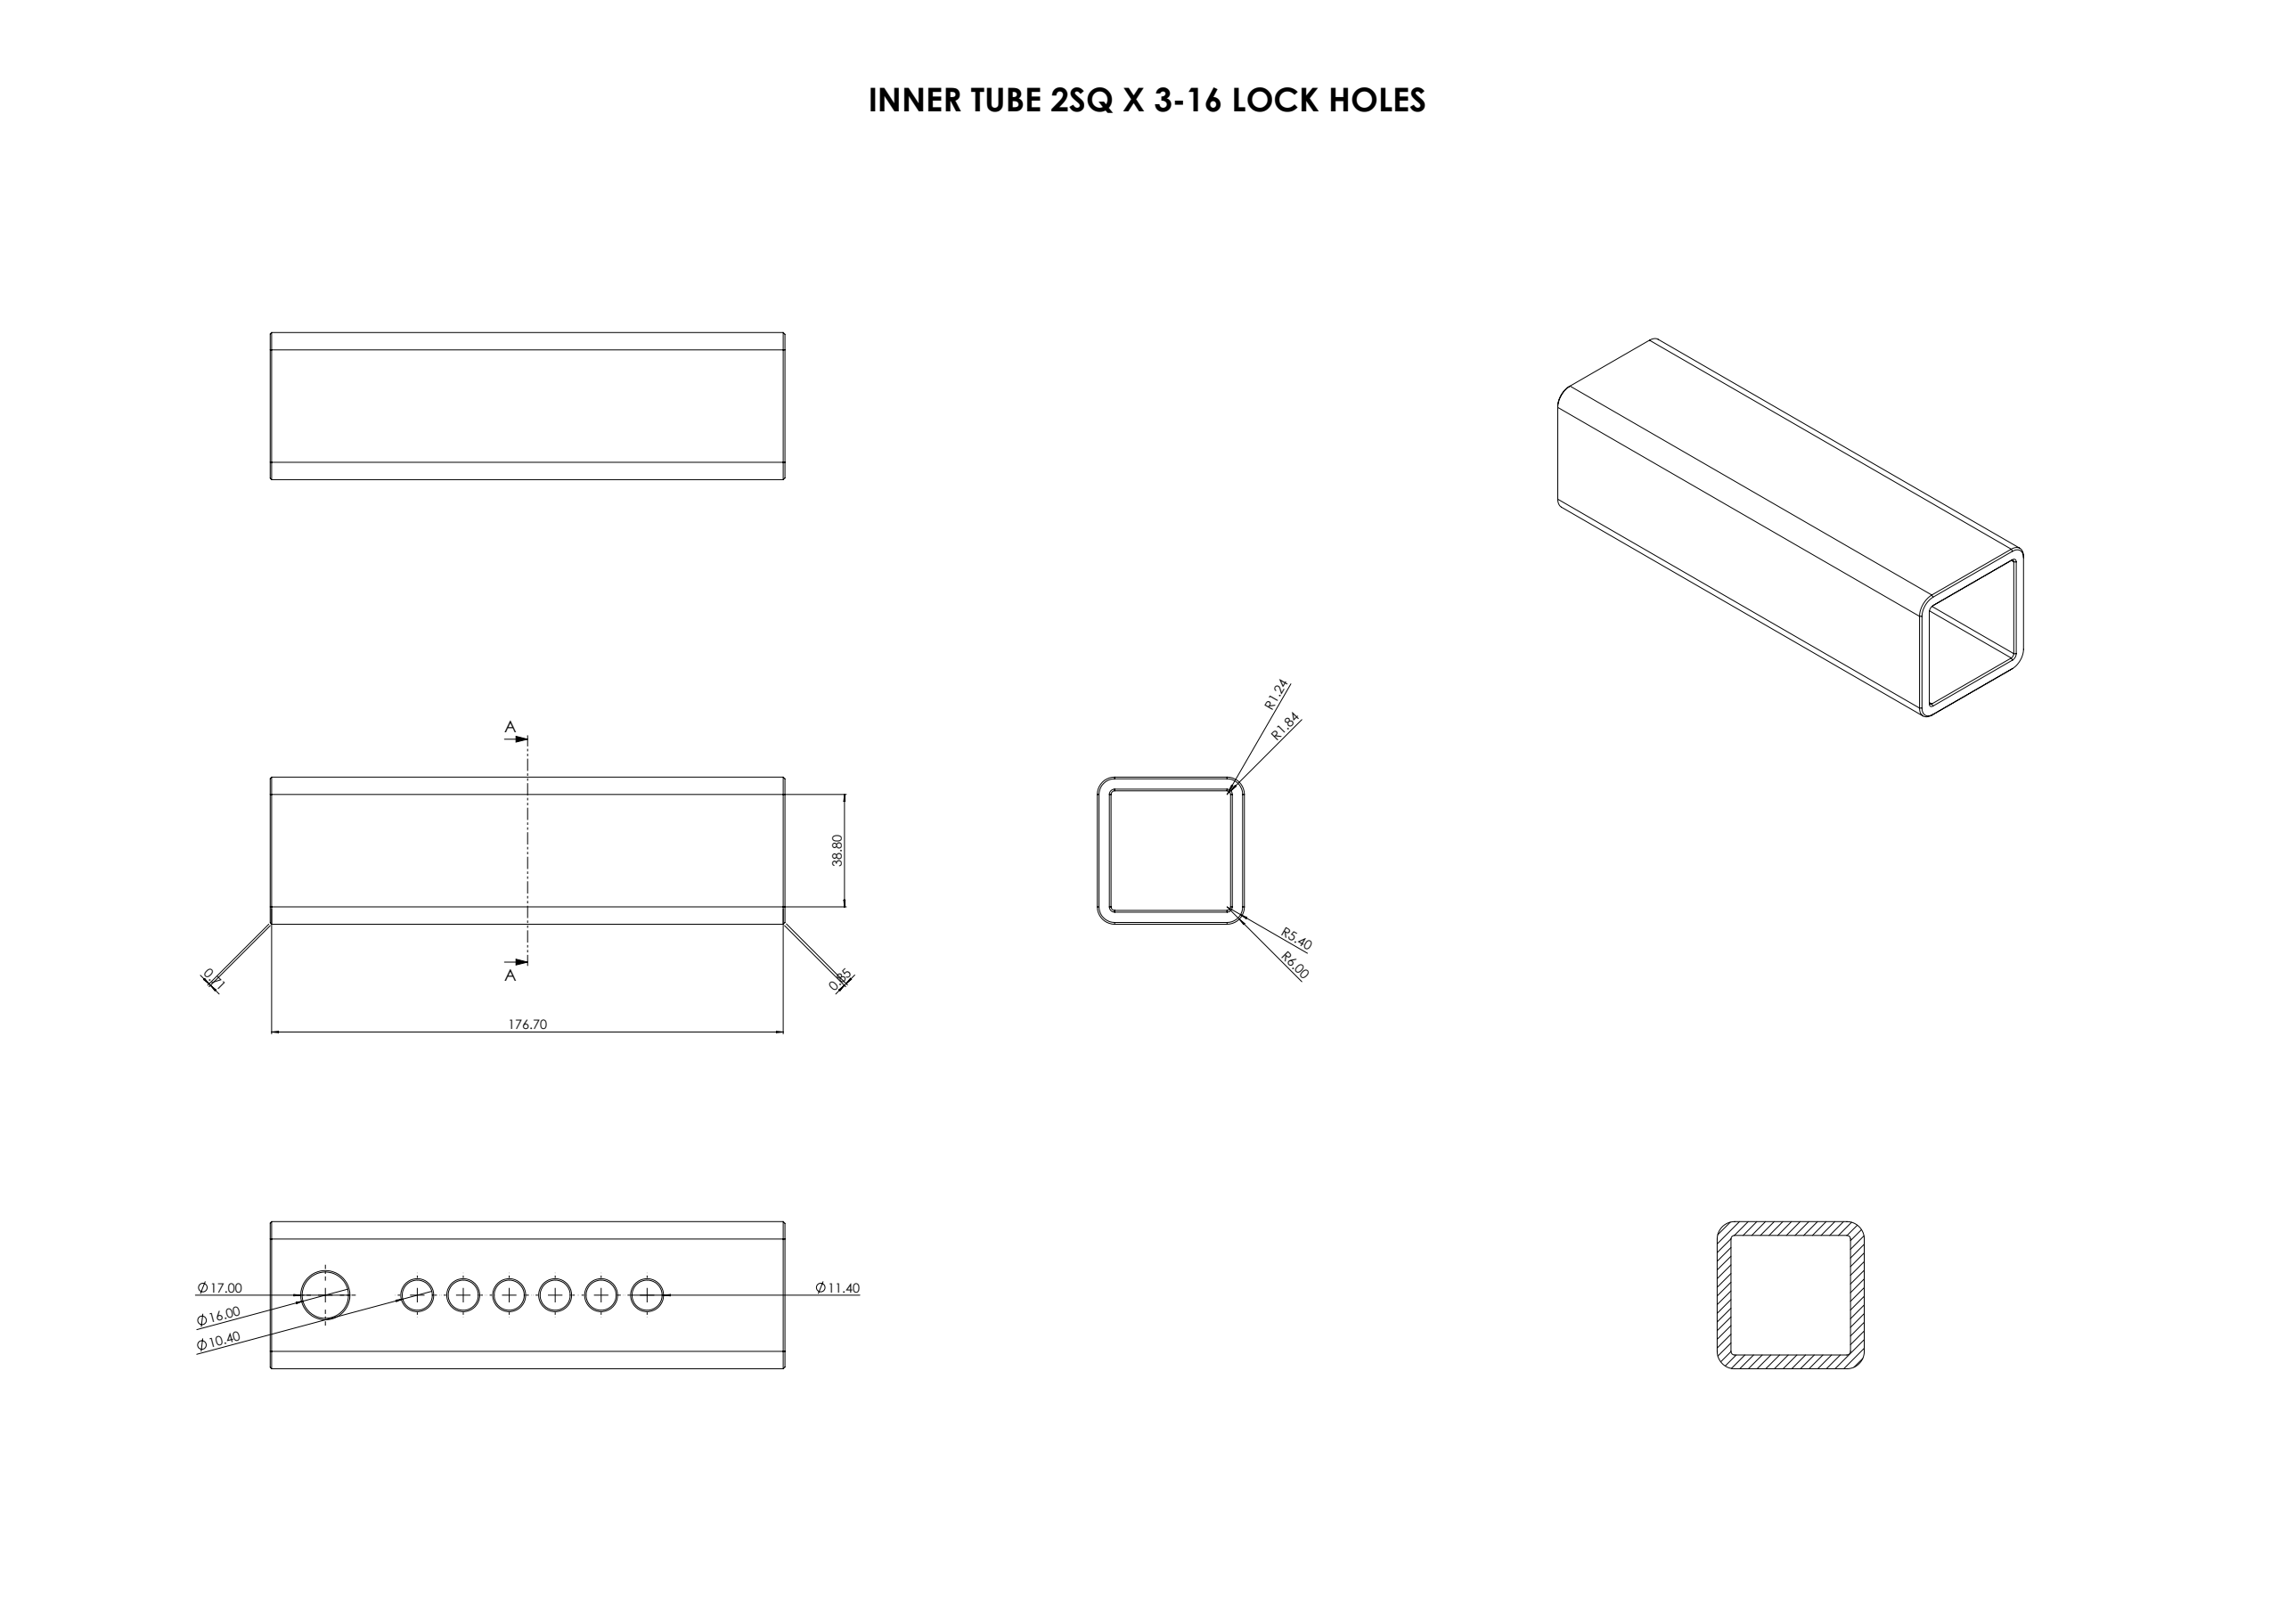
ISO-10303-21;
HEADER;
/* Generated by software containing ST-Developer
 * from STEP Tools, Inc. (www.steptools.com) 
 */

FILE_DESCRIPTION(
/* description */ (''),
/* implementation_level */ '2;1');

FILE_NAME(
/* name */ '05_Inner_Tube_2sq_x_3-16_Lock_Holes.step',
/* time_stamp */ '2026-10-25T01:30:15-07:00',
/* author */ (''),
/* organization */ (''),
/* preprocessor_version */ 'ST-DEVELOPER v20.2',
/* originating_system */ 'Autodesk Translation Framework v15.15.0.0',
/* authorisation */ '');

FILE_SCHEMA (('AUTOMOTIVE_DESIGN { 1 0 10303 214 3 1 1 }'));
ENDSEC;

DATA;
#10=MECHANICAL_DESIGN_GEOMETRIC_PRESENTATION_REPRESENTATION('',(#567),#32309);
#539=SHAPE_REPRESENTATION_RELATIONSHIP('SRR','None',#32366,#553);
#553=ADVANCED_BREP_SHAPE_REPRESENTATION('',(#581),#32299);
#567=STYLED_ITEM('',(#32488),#581);
#581=MANIFOLD_SOLID_BREP('Body1',#13808);
#599=FACE_BOUND('',#2235,.T.);
#600=FACE_BOUND('',#2236,.T.);
#601=FACE_BOUND('',#2237,.T.);
#602=FACE_BOUND('',#2238,.T.);
#603=FACE_BOUND('',#2239,.T.);
#604=FACE_BOUND('',#2240,.T.);
#605=FACE_BOUND('',#2254,.T.);
#606=FACE_BOUND('',#2255,.T.);
#607=FACE_BOUND('',#2256,.T.);
#608=FACE_BOUND('',#2257,.T.);
#609=FACE_BOUND('',#2258,.T.);
#610=FACE_BOUND('',#2259,.T.);
#611=FACE_BOUND('',#2260,.T.);
#612=FACE_BOUND('',#2273,.T.);
#613=FACE_BOUND('',#2288,.T.);
#614=FACE_BOUND('',#2289,.T.);
#615=FACE_BOUND('',#2290,.T.);
#616=FACE_BOUND('',#2291,.T.);
#617=FACE_BOUND('',#2292,.T.);
#618=FACE_BOUND('',#2293,.T.);
#619=FACE_BOUND('',#2294,.T.);
#620=FACE_BOUND('',#2312,.T.);
#621=FACE_BOUND('',#2313,.T.);
#622=FACE_BOUND('',#2314,.T.);
#623=FACE_BOUND('',#2315,.T.);
#624=FACE_BOUND('',#2316,.T.);
#625=FACE_BOUND('',#2317,.T.);
#626=FACE_BOUND('',#2334,.T.);
#685=CYLINDRICAL_SURFACE('',#14214,5.2);
#686=CYLINDRICAL_SURFACE('',#14218,5.2);
#687=CYLINDRICAL_SURFACE('',#14222,5.2);
#688=CYLINDRICAL_SURFACE('',#14226,5.2);
#689=CYLINDRICAL_SURFACE('',#14230,5.2);
#690=CYLINDRICAL_SURFACE('',#14234,5.2);
#691=CYLINDRICAL_SURFACE('',#14246,5.2);
#692=CYLINDRICAL_SURFACE('',#14264,1.2375);
#693=CYLINDRICAL_SURFACE('',#14266,1.2375);
#694=CYLINDRICAL_SURFACE('',#14275,8.);
#695=CYLINDRICAL_SURFACE('',#14279,5.2);
#696=CYLINDRICAL_SURFACE('',#14283,5.2);
#697=CYLINDRICAL_SURFACE('',#14287,5.2);
#698=CYLINDRICAL_SURFACE('',#14291,5.2);
#699=CYLINDRICAL_SURFACE('',#14295,5.2);
#700=CYLINDRICAL_SURFACE('',#14324,6.00000000000001);
#701=CYLINDRICAL_SURFACE('',#14326,6.00000000000001);
#702=CYLINDRICAL_SURFACE('',#14355,6.00000000000001);
#703=CYLINDRICAL_SURFACE('',#14371,1.2375);
#704=CYLINDRICAL_SURFACE('',#14373,1.23749999999999);
#705=CYLINDRICAL_SURFACE('',#14376,6.00000000000001);
#855=CIRCLE('',#14206,5.69999999999999);
#856=CIRCLE('',#14207,5.2);
#857=CIRCLE('',#14209,5.7);
#858=CIRCLE('',#14210,5.7);
#859=CIRCLE('',#14211,5.69999999999999);
#860=CIRCLE('',#14212,5.7);
#861=CIRCLE('',#14213,5.7);
#862=CIRCLE('',#14215,5.2);
#863=CIRCLE('',#14217,5.2);
#864=CIRCLE('',#14219,5.2);
#865=CIRCLE('',#14221,5.2);
#866=CIRCLE('',#14223,5.2);
#867=CIRCLE('',#14225,5.2);
#868=CIRCLE('',#14227,5.2);
#869=CIRCLE('',#14229,5.2);
#870=CIRCLE('',#14231,5.2);
#871=CIRCLE('',#14233,5.2);
#872=CIRCLE('',#14235,5.2);
#873=CIRCLE('',#14237,5.69999999999999);
#874=CIRCLE('',#14238,5.2);
#875=CIRCLE('',#14240,5.7);
#876=CIRCLE('',#14241,5.7);
#877=CIRCLE('',#14242,5.69999999999999);
#878=CIRCLE('',#14243,5.7);
#879=CIRCLE('',#14244,5.7);
#880=CIRCLE('',#14245,8.5);
#881=CIRCLE('',#14247,5.2);
#882=CIRCLE('',#14250,1.2375);
#883=CIRCLE('',#14251,1.7375);
#884=CIRCLE('',#14254,1.23749999999999);
#885=CIRCLE('',#14255,1.7375);
#886=CIRCLE('',#14258,1.2375);
#887=CIRCLE('',#14259,1.7375);
#888=CIRCLE('',#14262,1.2375);
#889=CIRCLE('',#14263,1.7375);
#890=CIRCLE('',#14265,1.2375);
#891=CIRCLE('',#14267,1.2375);
#892=CIRCLE('',#14269,5.50000000000001);
#893=CIRCLE('',#14270,5.50000000000001);
#894=CIRCLE('',#14271,5.50000000000002);
#895=CIRCLE('',#14272,5.50000000000002);
#896=CIRCLE('',#14274,8.);
#897=CIRCLE('',#14276,8.);
#898=CIRCLE('',#14278,5.2);
#899=CIRCLE('',#14280,5.2);
#900=CIRCLE('',#14282,5.2);
#901=CIRCLE('',#14284,5.2);
#902=CIRCLE('',#14286,5.2);
#903=CIRCLE('',#14288,5.2);
#904=CIRCLE('',#14290,5.2);
#905=CIRCLE('',#14292,5.2);
#906=CIRCLE('',#14294,5.2);
#907=CIRCLE('',#14296,5.2);
#908=CIRCLE('',#14298,8.5);
#909=CIRCLE('',#14300,5.69999999999999);
#910=CIRCLE('',#14301,5.7);
#911=CIRCLE('',#14302,5.7);
#912=CIRCLE('',#14303,5.69999999999999);
#913=CIRCLE('',#14304,5.7);
#914=CIRCLE('',#14305,5.7);
#915=CIRCLE('',#14314,6.00000000000001);
#916=CIRCLE('',#14317,6.00000000000001);
#917=CIRCLE('',#14320,6.00000000000001);
#918=CIRCLE('',#14323,6.00000000000001);
#919=CIRCLE('',#14325,6.00000000000001);
#920=CIRCLE('',#14327,6.00000000000001);
#921=CIRCLE('',#14329,5.69999999999999);
#922=CIRCLE('',#14330,5.7);
#923=CIRCLE('',#14331,5.7);
#924=CIRCLE('',#14332,5.69999999999999);
#925=CIRCLE('',#14333,5.7);
#926=CIRCLE('',#14334,5.7);
#927=CIRCLE('',#14343,5.40000000000001);
#928=CIRCLE('',#14346,5.40000000000002);
#929=CIRCLE('',#14347,6.00000000000001);
#930=CIRCLE('',#14350,5.40000000000002);
#931=CIRCLE('',#14351,6.00000000000001);
#932=CIRCLE('',#14354,5.40000000000001);
#933=CIRCLE('',#14357,1.8375);
#934=CIRCLE('',#14358,1.8375);
#935=CIRCLE('',#14359,1.83749999999999);
#936=CIRCLE('',#14360,1.8375);
#937=CIRCLE('',#14365,1.2375);
#938=CIRCLE('',#14368,1.23749999999999);
#1135=CONICAL_SURFACE('',#14205,5.44999999999999,0.785398163397448);
#1136=CONICAL_SURFACE('',#14216,5.45,0.785398163397451);
#1137=CONICAL_SURFACE('',#14220,5.45,0.785398163397451);
#1138=CONICAL_SURFACE('',#14224,5.45,0.785398163397448);
#1139=CONICAL_SURFACE('',#14228,5.45,0.785398163397448);
#1140=CONICAL_SURFACE('',#14232,5.44999999999999,0.785398163397448);
#1141=CONICAL_SURFACE('',#14236,5.44999999999999,0.785398163397446);
#1142=CONICAL_SURFACE('',#14249,1.4875,0.785398163397449);
#1143=CONICAL_SURFACE('',#14253,1.48749999999999,0.785398163397452);
#1144=CONICAL_SURFACE('',#14257,1.4875,0.785398163397449);
#1145=CONICAL_SURFACE('',#14261,1.4875,0.785398163397449);
#1146=CONICAL_SURFACE('',#14273,8.25,0.785398163397446);
#1147=CONICAL_SURFACE('',#14277,5.45,0.785398163397446);
#1148=CONICAL_SURFACE('',#14281,5.45,0.785398163397446);
#1149=CONICAL_SURFACE('',#14285,5.45,0.785398163397448);
#1150=CONICAL_SURFACE('',#14289,5.45,0.785398163397448);
#1151=CONICAL_SURFACE('',#14293,5.44999999999999,0.785398163397446);
#1152=CONICAL_SURFACE('',#14297,8.25,0.785398163397446);
#1153=CONICAL_SURFACE('',#14306,5.44999999999999,0.785398163397446);
#1154=CONICAL_SURFACE('',#14307,5.45,0.785398163397446);
#1155=CONICAL_SURFACE('',#14308,5.45,0.785398163397446);
#1156=CONICAL_SURFACE('',#14309,5.45,0.785398163397448);
#1157=CONICAL_SURFACE('',#14310,5.45,0.785398163397448);
#1158=CONICAL_SURFACE('',#14311,5.44999999999999,0.785398163397446);
#1159=CONICAL_SURFACE('',#14313,5.75000000000002,0.785398163397449);
#1160=CONICAL_SURFACE('',#14316,5.75000000000002,0.785398163397449);
#1161=CONICAL_SURFACE('',#14319,5.75000000000001,0.785398163397451);
#1162=CONICAL_SURFACE('',#14322,5.75000000000001,0.785398163397449);
#1163=CONICAL_SURFACE('',#14335,5.44999999999999,0.785398163397448);
#1164=CONICAL_SURFACE('',#14336,5.45,0.785398163397448);
#1165=CONICAL_SURFACE('',#14337,5.45,0.785398163397448);
#1166=CONICAL_SURFACE('',#14338,5.45,0.785398163397451);
#1167=CONICAL_SURFACE('',#14339,5.45,0.785398163397451);
#1168=CONICAL_SURFACE('',#14340,5.44999999999999,0.785398163397448);
#1169=CONICAL_SURFACE('',#14342,5.70000000000001,0.785398163397431);
#1170=CONICAL_SURFACE('',#14345,5.70000000000002,0.785398163397426);
#1171=CONICAL_SURFACE('',#14349,5.70000000000002,0.785398163397426);
#1172=CONICAL_SURFACE('',#14353,5.70000000000001,0.785398163397431);
#1173=CONICAL_SURFACE('',#14362,1.5375,0.78539816339743);
#1174=CONICAL_SURFACE('',#14364,1.5375,0.78539816339743);
#1175=CONICAL_SURFACE('',#14367,1.53749999999999,0.785398163397429);
#1176=CONICAL_SURFACE('',#14370,1.5375,0.785398163397426);
#1426=FACE_OUTER_BOUND('',#2233,.T.);
#1427=FACE_OUTER_BOUND('',#2234,.T.);
#1428=FACE_OUTER_BOUND('',#2241,.T.);
#1429=FACE_OUTER_BOUND('',#2242,.T.);
#1430=FACE_OUTER_BOUND('',#2243,.T.);
#1431=FACE_OUTER_BOUND('',#2244,.T.);
#1432=FACE_OUTER_BOUND('',#2245,.T.);
#1433=FACE_OUTER_BOUND('',#2246,.T.);
#1434=FACE_OUTER_BOUND('',#2247,.T.);
#1435=FACE_OUTER_BOUND('',#2248,.T.);
#1436=FACE_OUTER_BOUND('',#2249,.T.);
#1437=FACE_OUTER_BOUND('',#2250,.T.);
#1438=FACE_OUTER_BOUND('',#2251,.T.);
#1439=FACE_OUTER_BOUND('',#2252,.T.);
#1440=FACE_OUTER_BOUND('',#2253,.T.);
#1441=FACE_OUTER_BOUND('',#2261,.T.);
#1442=FACE_OUTER_BOUND('',#2262,.T.);
#1443=FACE_OUTER_BOUND('',#2263,.T.);
#1444=FACE_OUTER_BOUND('',#2264,.T.);
#1445=FACE_OUTER_BOUND('',#2265,.T.);
#1446=FACE_OUTER_BOUND('',#2266,.T.);
#1447=FACE_OUTER_BOUND('',#2267,.T.);
#1448=FACE_OUTER_BOUND('',#2268,.T.);
#1449=FACE_OUTER_BOUND('',#2269,.T.);
#1450=FACE_OUTER_BOUND('',#2270,.T.);
#1451=FACE_OUTER_BOUND('',#2271,.T.);
#1452=FACE_OUTER_BOUND('',#2272,.T.);
#1453=FACE_OUTER_BOUND('',#2274,.T.);
#1454=FACE_OUTER_BOUND('',#2275,.T.);
#1455=FACE_OUTER_BOUND('',#2276,.T.);
#1456=FACE_OUTER_BOUND('',#2277,.T.);
#1457=FACE_OUTER_BOUND('',#2278,.T.);
#1458=FACE_OUTER_BOUND('',#2279,.T.);
#1459=FACE_OUTER_BOUND('',#2280,.T.);
#1460=FACE_OUTER_BOUND('',#2281,.T.);
#1461=FACE_OUTER_BOUND('',#2282,.T.);
#1462=FACE_OUTER_BOUND('',#2283,.T.);
#1463=FACE_OUTER_BOUND('',#2284,.T.);
#1464=FACE_OUTER_BOUND('',#2285,.T.);
#1465=FACE_OUTER_BOUND('',#2286,.T.);
#1466=FACE_OUTER_BOUND('',#2287,.T.);
#1467=FACE_OUTER_BOUND('',#2295,.T.);
#1468=FACE_OUTER_BOUND('',#2296,.T.);
#1469=FACE_OUTER_BOUND('',#2297,.T.);
#1470=FACE_OUTER_BOUND('',#2298,.T.);
#1471=FACE_OUTER_BOUND('',#2299,.T.);
#1472=FACE_OUTER_BOUND('',#2300,.T.);
#1473=FACE_OUTER_BOUND('',#2301,.T.);
#1474=FACE_OUTER_BOUND('',#2302,.T.);
#1475=FACE_OUTER_BOUND('',#2303,.T.);
#1476=FACE_OUTER_BOUND('',#2304,.T.);
#1477=FACE_OUTER_BOUND('',#2305,.T.);
#1478=FACE_OUTER_BOUND('',#2306,.T.);
#1479=FACE_OUTER_BOUND('',#2307,.T.);
#1480=FACE_OUTER_BOUND('',#2308,.T.);
#1481=FACE_OUTER_BOUND('',#2309,.T.);
#1482=FACE_OUTER_BOUND('',#2310,.T.);
#1483=FACE_OUTER_BOUND('',#2311,.T.);
#1484=FACE_OUTER_BOUND('',#2318,.T.);
#1485=FACE_OUTER_BOUND('',#2319,.T.);
#1486=FACE_OUTER_BOUND('',#2320,.T.);
#1487=FACE_OUTER_BOUND('',#2321,.T.);
#1488=FACE_OUTER_BOUND('',#2322,.T.);
#1489=FACE_OUTER_BOUND('',#2323,.T.);
#1490=FACE_OUTER_BOUND('',#2324,.T.);
#1491=FACE_OUTER_BOUND('',#2325,.T.);
#1492=FACE_OUTER_BOUND('',#2326,.T.);
#1493=FACE_OUTER_BOUND('',#2327,.T.);
#1494=FACE_OUTER_BOUND('',#2328,.T.);
#1495=FACE_OUTER_BOUND('',#2329,.T.);
#1496=FACE_OUTER_BOUND('',#2330,.T.);
#1497=FACE_OUTER_BOUND('',#2331,.T.);
#1498=FACE_OUTER_BOUND('',#2332,.T.);
#1499=FACE_OUTER_BOUND('',#2333,.T.);
#1500=FACE_OUTER_BOUND('',#2335,.T.);
#1501=FACE_OUTER_BOUND('',#2336,.T.);
#1502=FACE_OUTER_BOUND('',#2337,.T.);
#1503=FACE_OUTER_BOUND('',#2338,.T.);
#1504=FACE_OUTER_BOUND('',#2339,.T.);
#1505=FACE_OUTER_BOUND('',#2340,.T.);
#1506=FACE_OUTER_BOUND('',#2341,.T.);
#1507=FACE_OUTER_BOUND('',#2342,.T.);
#1508=FACE_OUTER_BOUND('',#2343,.T.);
#1509=FACE_OUTER_BOUND('',#2344,.T.);
#1510=FACE_OUTER_BOUND('',#2345,.T.);
#1511=FACE_OUTER_BOUND('',#2346,.T.);
#1512=FACE_OUTER_BOUND('',#2347,.T.);
#1513=FACE_OUTER_BOUND('',#2348,.T.);
#1514=FACE_OUTER_BOUND('',#2349,.T.);
#2233=EDGE_LOOP('',(#9555,#9556,#9557,#9558));
#2234=EDGE_LOOP('',(#9559,#9560,#9561,#9562));
#2235=EDGE_LOOP('',(#9563));
#2236=EDGE_LOOP('',(#9564));
#2237=EDGE_LOOP('',(#9565));
#2238=EDGE_LOOP('',(#9566));
#2239=EDGE_LOOP('',(#9567));
#2240=EDGE_LOOP('',(#9568));
#2241=EDGE_LOOP('',(#9569,#9570,#9571,#9572));
#2242=EDGE_LOOP('',(#9573,#9574,#9575,#9576));
#2243=EDGE_LOOP('',(#9577,#9578,#9579,#9580));
#2244=EDGE_LOOP('',(#9581,#9582,#9583,#9584));
#2245=EDGE_LOOP('',(#9585,#9586,#9587,#9588));
#2246=EDGE_LOOP('',(#9589,#9590,#9591,#9592));
#2247=EDGE_LOOP('',(#9593,#9594,#9595,#9596));
#2248=EDGE_LOOP('',(#9597,#9598,#9599,#9600));
#2249=EDGE_LOOP('',(#9601,#9602,#9603,#9604));
#2250=EDGE_LOOP('',(#9605,#9606,#9607,#9608));
#2251=EDGE_LOOP('',(#9609,#9610,#9611,#9612));
#2252=EDGE_LOOP('',(#9613,#9614,#9615,#9616));
#2253=EDGE_LOOP('',(#9617,#9618,#9619,#9620));
#2254=EDGE_LOOP('',(#9621));
#2255=EDGE_LOOP('',(#9622));
#2256=EDGE_LOOP('',(#9623));
#2257=EDGE_LOOP('',(#9624));
#2258=EDGE_LOOP('',(#9625));
#2259=EDGE_LOOP('',(#9626));
#2260=EDGE_LOOP('',(#9627));
#2261=EDGE_LOOP('',(#9628,#9629,#9630,#9631));
#2262=EDGE_LOOP('',(#9632,#9633,#9634,#9635));
#2263=EDGE_LOOP('',(#9636,#9637,#9638,#9639));
#2264=EDGE_LOOP('',(#9640,#9641,#9642,#9643));
#2265=EDGE_LOOP('',(#9644,#9645,#9646,#9647));
#2266=EDGE_LOOP('',(#9648,#9649,#9650,#9651));
#2267=EDGE_LOOP('',(#9652,#9653,#9654,#9655));
#2268=EDGE_LOOP('',(#9656,#9657,#9658,#9659));
#2269=EDGE_LOOP('',(#9660,#9661,#9662,#9663));
#2270=EDGE_LOOP('',(#9664,#9665,#9666,#9667));
#2271=EDGE_LOOP('',(#9668,#9669,#9670,#9671));
#2272=EDGE_LOOP('',(#9672,#9673,#9674,#9675,#9676,#9677,#9678,#9679));
#2273=EDGE_LOOP('',(#9680,#9681,#9682,#9683,#9684,#9685,#9686,#9687));
#2274=EDGE_LOOP('',(#9688,#9689,#9690,#9691));
#2275=EDGE_LOOP('',(#9692,#9693,#9694,#9695));
#2276=EDGE_LOOP('',(#9696,#9697,#9698,#9699));
#2277=EDGE_LOOP('',(#9700,#9701,#9702,#9703));
#2278=EDGE_LOOP('',(#9704,#9705,#9706,#9707));
#2279=EDGE_LOOP('',(#9708,#9709,#9710,#9711));
#2280=EDGE_LOOP('',(#9712,#9713,#9714,#9715));
#2281=EDGE_LOOP('',(#9716,#9717,#9718,#9719));
#2282=EDGE_LOOP('',(#9720,#9721,#9722,#9723));
#2283=EDGE_LOOP('',(#9724,#9725,#9726,#9727));
#2284=EDGE_LOOP('',(#9728,#9729,#9730,#9731));
#2285=EDGE_LOOP('',(#9732,#9733,#9734,#9735));
#2286=EDGE_LOOP('',(#9736,#9737,#9738,#9739));
#2287=EDGE_LOOP('',(#9740,#9741,#9742,#9743));
#2288=EDGE_LOOP('',(#9744));
#2289=EDGE_LOOP('',(#9745));
#2290=EDGE_LOOP('',(#9746));
#2291=EDGE_LOOP('',(#9747));
#2292=EDGE_LOOP('',(#9748));
#2293=EDGE_LOOP('',(#9749));
#2294=EDGE_LOOP('',(#9750));
#2295=EDGE_LOOP('',(#9751,#9752,#9753,#9754));
#2296=EDGE_LOOP('',(#9755,#9756,#9757,#9758));
#2297=EDGE_LOOP('',(#9759,#9760,#9761,#9762));
#2298=EDGE_LOOP('',(#9763,#9764,#9765,#9766));
#2299=EDGE_LOOP('',(#9767,#9768,#9769,#9770));
#2300=EDGE_LOOP('',(#9771,#9772,#9773,#9774));
#2301=EDGE_LOOP('',(#9775,#9776,#9777,#9778));
#2302=EDGE_LOOP('',(#9779,#9780,#9781,#9782));
#2303=EDGE_LOOP('',(#9783,#9784,#9785,#9786));
#2304=EDGE_LOOP('',(#9787,#9788,#9789,#9790));
#2305=EDGE_LOOP('',(#9791,#9792,#9793,#9794));
#2306=EDGE_LOOP('',(#9795,#9796,#9797,#9798));
#2307=EDGE_LOOP('',(#9799,#9800,#9801,#9802));
#2308=EDGE_LOOP('',(#9803,#9804,#9805,#9806));
#2309=EDGE_LOOP('',(#9807,#9808,#9809,#9810));
#2310=EDGE_LOOP('',(#9811,#9812,#9813,#9814));
#2311=EDGE_LOOP('',(#9815,#9816,#9817,#9818));
#2312=EDGE_LOOP('',(#9819));
#2313=EDGE_LOOP('',(#9820));
#2314=EDGE_LOOP('',(#9821));
#2315=EDGE_LOOP('',(#9822));
#2316=EDGE_LOOP('',(#9823));
#2317=EDGE_LOOP('',(#9824));
#2318=EDGE_LOOP('',(#9825,#9826,#9827,#9828));
#2319=EDGE_LOOP('',(#9829,#9830,#9831,#9832));
#2320=EDGE_LOOP('',(#9833,#9834,#9835,#9836));
#2321=EDGE_LOOP('',(#9837,#9838,#9839,#9840));
#2322=EDGE_LOOP('',(#9841,#9842,#9843,#9844));
#2323=EDGE_LOOP('',(#9845,#9846,#9847,#9848));
#2324=EDGE_LOOP('',(#9849,#9850,#9851,#9852));
#2325=EDGE_LOOP('',(#9853,#9854,#9855,#9856));
#2326=EDGE_LOOP('',(#9857,#9858,#9859,#9860));
#2327=EDGE_LOOP('',(#9861,#9862,#9863,#9864));
#2328=EDGE_LOOP('',(#9865,#9866,#9867,#9868));
#2329=EDGE_LOOP('',(#9869,#9870,#9871,#9872));
#2330=EDGE_LOOP('',(#9873,#9874,#9875,#9876));
#2331=EDGE_LOOP('',(#9877,#9878,#9879,#9880));
#2332=EDGE_LOOP('',(#9881,#9882,#9883,#9884));
#2333=EDGE_LOOP('',(#9885,#9886,#9887,#9888,#9889,#9890,#9891,#9892));
#2334=EDGE_LOOP('',(#9893,#9894,#9895,#9896,#9897,#9898,#9899,#9900));
#2335=EDGE_LOOP('',(#9901,#9902,#9903,#9904));
#2336=EDGE_LOOP('',(#9905,#9906,#9907,#9908));
#2337=EDGE_LOOP('',(#9909,#9910,#9911,#9912));
#2338=EDGE_LOOP('',(#9913,#9914,#9915,#9916));
#2339=EDGE_LOOP('',(#9917,#9918,#9919,#9920));
#2340=EDGE_LOOP('',(#9921,#9922,#9923,#9924));
#2341=EDGE_LOOP('',(#9925,#9926,#9927,#9928));
#2342=EDGE_LOOP('',(#9929,#9930,#9931,#9932));
#2343=EDGE_LOOP('',(#9933,#9934,#9935,#9936));
#2344=EDGE_LOOP('',(#9937,#9938,#9939,#9940));
#2345=EDGE_LOOP('',(#9941,#9942,#9943,#9944));
#2346=EDGE_LOOP('',(#9945,#9946,#9947,#9948));
#2347=EDGE_LOOP('',(#9949,#9950,#9951,#9952));
#2348=EDGE_LOOP('',(#9953,#9954,#9955,#9956));
#2349=EDGE_LOOP('',(#9957,#9958,#9959,#9960));
#3148=LINE('',#22237,#4459);
#3149=LINE('',#22242,#4460);
#3150=LINE('',#22244,#4461);
#3151=LINE('',#22246,#4462);
#3152=LINE('',#22247,#4463);
#3153=LINE('',#22261,#4464);
#3154=LINE('',#22264,#4465);
#3155=LINE('',#22269,#4466);
#3156=LINE('',#22272,#4467);
#3157=LINE('',#22277,#4468);
#3158=LINE('',#22280,#4469);
#3159=LINE('',#22285,#4470);
#3160=LINE('',#22288,#4471);
#3161=LINE('',#22293,#4472);
#3162=LINE('',#22296,#4473);
#3163=LINE('',#22301,#4474);
#3164=LINE('',#22306,#4475);
#3165=LINE('',#22311,#4476);
#3166=LINE('',#22313,#4477);
#3167=LINE('',#22315,#4478);
#3168=LINE('',#22316,#4479);
#3169=LINE('',#22332,#4480);
#3170=LINE('',#22335,#4481);
#3171=LINE('',#22337,#4482);
#3172=LINE('',#22338,#4483);
#3173=LINE('',#22342,#4484);
#3174=LINE('',#22348,#4485);
#3175=LINE('',#22349,#4486);
#3176=LINE('',#22350,#4487);
#3177=LINE('',#22354,#4488);
#3178=LINE('',#22360,#4489);
#3179=LINE('',#22361,#4490);
#3180=LINE('',#22362,#4491);
#3181=LINE('',#22365,#4492);
#3182=LINE('',#22370,#4493);
#3183=LINE('',#22371,#4494);
#3184=LINE('',#22378,#4495);
#3185=LINE('',#22384,#4496);
#3186=LINE('',#22388,#4497);
#3187=LINE('',#22392,#4498);
#3188=LINE('',#22396,#4499);
#3189=LINE('',#22400,#4500);
#3190=LINE('',#22405,#4501);
#3191=LINE('',#22408,#4502);
#3192=LINE('',#22413,#4503);
#3193=LINE('',#22416,#4504);
#3194=LINE('',#22421,#4505);
#3195=LINE('',#22424,#4506);
#3196=LINE('',#22429,#4507);
#3197=LINE('',#22432,#4508);
#3198=LINE('',#22437,#4509);
#3199=LINE('',#22440,#4510);
#3200=LINE('',#22445,#4511);
#3201=LINE('',#22449,#4512);
#3202=LINE('',#22453,#4513);
#3203=LINE('',#22455,#4514);
#3204=LINE('',#22457,#4515);
#3205=LINE('',#22458,#4516);
#3206=LINE('',#22472,#4517);
#3207=LINE('',#22474,#4518);
#3208=LINE('',#22476,#4519);
#3209=LINE('',#22478,#4520);
#3210=LINE('',#22480,#4521);
#3211=LINE('',#22482,#4522);
#3212=LINE('',#22485,#4523);
#3213=LINE('',#22487,#4524);
#3214=LINE('',#22488,#4525);
#3215=LINE('',#22491,#4526);
#3216=LINE('',#22495,#4527);
#3217=LINE('',#22496,#4528);
#3218=LINE('',#22499,#4529);
#3219=LINE('',#22503,#4530);
#3220=LINE('',#22504,#4531);
#3221=LINE('',#22506,#4532);
#3222=LINE('',#22509,#4533);
#3223=LINE('',#22515,#4534);
#3224=LINE('',#22518,#4535);
#3225=LINE('',#22522,#4536);
#3226=LINE('',#22523,#4537);
#3227=LINE('',#22537,#4538);
#3228=LINE('',#22539,#4539);
#3229=LINE('',#22541,#4540);
#3230=LINE('',#22543,#4541);
#3231=LINE('',#22545,#4542);
#3232=LINE('',#22547,#4543);
#3233=LINE('',#22550,#4544);
#3234=LINE('',#22552,#4545);
#3235=LINE('',#22553,#4546);
#3236=LINE('',#22556,#4547);
#3237=LINE('',#22560,#4548);
#3238=LINE('',#22561,#4549);
#3239=LINE('',#22565,#4550);
#3240=LINE('',#22571,#4551);
#3241=LINE('',#22572,#4552);
#3242=LINE('',#22573,#4553);
#3243=LINE('',#22577,#4554);
#3244=LINE('',#22582,#4555);
#3245=LINE('',#22583,#4556);
#3246=LINE('',#22584,#4557);
#3247=LINE('',#22588,#4558);
#3248=LINE('',#22592,#4559);
#3249=LINE('',#22596,#4560);
#3250=LINE('',#22600,#4561);
#3251=LINE('',#22604,#4562);
#3252=LINE('',#22607,#4563);
#3253=LINE('',#22608,#4564);
#3254=LINE('',#22610,#4565);
#3255=LINE('',#22612,#4566);
#3256=LINE('',#22615,#4567);
#3257=LINE('',#22619,#4568);
#3258=LINE('',#22620,#4569);
#3259=LINE('',#22623,#4570);
#3260=LINE('',#22626,#4571);
#3261=LINE('',#22627,#4572);
#3262=LINE('',#22630,#4573);
#3263=LINE('',#22632,#4574);
#3264=LINE('',#22634,#4575);
#3265=LINE('',#22637,#4576);
#3266=LINE('',#22639,#4577);
#4459=VECTOR('',#15724,5.45);
#4460=VECTOR('',#15729,10.);
#4461=VECTOR('',#15730,10.);
#4462=VECTOR('',#15731,10.);
#4463=VECTOR('',#15732,10.);
#4464=VECTOR('',#15747,5.2);
#4465=VECTOR('',#15750,5.45);
#4466=VECTOR('',#15757,5.2);
#4467=VECTOR('',#15760,5.45);
#4468=VECTOR('',#15767,5.2);
#4469=VECTOR('',#15770,5.45);
#4470=VECTOR('',#15777,5.2);
#4471=VECTOR('',#15780,5.45);
#4472=VECTOR('',#15787,5.2);
#4473=VECTOR('',#15790,5.45);
#4474=VECTOR('',#15797,5.2);
#4475=VECTOR('',#15802,5.45);
#4476=VECTOR('',#15807,10.);
#4477=VECTOR('',#15808,10.);
#4478=VECTOR('',#15809,10.);
#4479=VECTOR('',#15810,10.);
#4480=VECTOR('',#15827,5.2);
#4481=VECTOR('',#15830,10.);
#4482=VECTOR('',#15831,10.);
#4483=VECTOR('',#15832,10.);
#4484=VECTOR('',#15835,10.);
#4485=VECTOR('',#15842,10.);
#4486=VECTOR('',#15843,10.);
#4487=VECTOR('',#15844,10.);
#4488=VECTOR('',#15847,10.);
#4489=VECTOR('',#15854,10.);
#4490=VECTOR('',#15855,10.);
#4491=VECTOR('',#15856,10.);
#4492=VECTOR('',#15859,10.);
#4493=VECTOR('',#15866,10.);
#4494=VECTOR('',#15867,10.);
#4495=VECTOR('',#15878,10.);
#4496=VECTOR('',#15885,10.);
#4497=VECTOR('',#15888,10.);
#4498=VECTOR('',#15891,10.);
#4499=VECTOR('',#15894,10.);
#4500=VECTOR('',#15899,8.25);
#4501=VECTOR('',#15906,8.);
#4502=VECTOR('',#15909,5.45);
#4503=VECTOR('',#15916,5.2);
#4504=VECTOR('',#15919,5.45);
#4505=VECTOR('',#15926,5.2);
#4506=VECTOR('',#15929,5.45);
#4507=VECTOR('',#15936,5.2);
#4508=VECTOR('',#15939,5.45);
#4509=VECTOR('',#15946,5.2);
#4510=VECTOR('',#15949,5.45);
#4511=VECTOR('',#15956,5.2);
#4512=VECTOR('',#15961,8.25);
#4513=VECTOR('',#15964,10.);
#4514=VECTOR('',#15965,10.);
#4515=VECTOR('',#15966,10.);
#4516=VECTOR('',#15967,10.);
#4517=VECTOR('',#15982,5.45);
#4518=VECTOR('',#15985,5.45);
#4519=VECTOR('',#15988,5.45);
#4520=VECTOR('',#15991,5.45);
#4521=VECTOR('',#15994,5.45);
#4522=VECTOR('',#15997,5.45);
#4523=VECTOR('',#16000,10.);
#4524=VECTOR('',#16001,10.);
#4525=VECTOR('',#16002,10.);
#4526=VECTOR('',#16005,10.);
#4527=VECTOR('',#16010,10.);
#4528=VECTOR('',#16011,10.);
#4529=VECTOR('',#16014,10.);
#4530=VECTOR('',#16019,10.);
#4531=VECTOR('',#16020,10.);
#4532=VECTOR('',#16023,10.);
#4533=VECTOR('',#16028,10.);
#4534=VECTOR('',#16037,10.);
#4535=VECTOR('',#16040,10.);
#4536=VECTOR('',#16045,10.);
#4537=VECTOR('',#16046,10.);
#4538=VECTOR('',#16061,5.45);
#4539=VECTOR('',#16064,5.45);
#4540=VECTOR('',#16067,5.45);
#4541=VECTOR('',#16070,5.45);
#4542=VECTOR('',#16073,5.45);
#4543=VECTOR('',#16076,5.45);
#4544=VECTOR('',#16079,10.);
#4545=VECTOR('',#16080,10.);
#4546=VECTOR('',#16081,10.);
#4547=VECTOR('',#16084,10.);
#4548=VECTOR('',#16089,10.);
#4549=VECTOR('',#16090,10.);
#4550=VECTOR('',#16093,10.);
#4551=VECTOR('',#16100,10.);
#4552=VECTOR('',#16101,10.);
#4553=VECTOR('',#16102,10.);
#4554=VECTOR('',#16105,10.);
#4555=VECTOR('',#16112,10.);
#4556=VECTOR('',#16113,10.);
#4557=VECTOR('',#16114,10.);
#4558=VECTOR('',#16121,10.);
#4559=VECTOR('',#16124,10.);
#4560=VECTOR('',#16127,10.);
#4561=VECTOR('',#16130,10.);
#4562=VECTOR('',#16133,10.);
#4563=VECTOR('',#16138,10.);
#4564=VECTOR('',#16139,10.);
#4565=VECTOR('',#16142,10.);
#4566=VECTOR('',#16145,10.);
#4567=VECTOR('',#16148,10.);
#4568=VECTOR('',#16153,10.);
#4569=VECTOR('',#16154,10.);
#4570=VECTOR('',#16157,10.);
#4571=VECTOR('',#16162,10.);
#4572=VECTOR('',#16163,10.);
#4573=VECTOR('',#16168,10.);
#4574=VECTOR('',#16171,10.);
#4575=VECTOR('',#16174,10.);
#4576=VECTOR('',#16179,10.);
#4577=VECTOR('',#16182,10.);
#5780=VERTEX_POINT('',#22234);
#5781=VERTEX_POINT('',#22236);
#5782=VERTEX_POINT('',#22240);
#5783=VERTEX_POINT('',#22241);
#5784=VERTEX_POINT('',#22243);
#5785=VERTEX_POINT('',#22245);
#5786=VERTEX_POINT('',#22248);
#5787=VERTEX_POINT('',#22250);
#5788=VERTEX_POINT('',#22252);
#5789=VERTEX_POINT('',#22254);
#5790=VERTEX_POINT('',#22256);
#5791=VERTEX_POINT('',#22259);
#5792=VERTEX_POINT('',#22263);
#5793=VERTEX_POINT('',#22267);
#5794=VERTEX_POINT('',#22271);
#5795=VERTEX_POINT('',#22275);
#5796=VERTEX_POINT('',#22279);
#5797=VERTEX_POINT('',#22283);
#5798=VERTEX_POINT('',#22287);
#5799=VERTEX_POINT('',#22291);
#5800=VERTEX_POINT('',#22295);
#5801=VERTEX_POINT('',#22299);
#5802=VERTEX_POINT('',#22303);
#5803=VERTEX_POINT('',#22305);
#5804=VERTEX_POINT('',#22309);
#5805=VERTEX_POINT('',#22310);
#5806=VERTEX_POINT('',#22312);
#5807=VERTEX_POINT('',#22314);
#5808=VERTEX_POINT('',#22317);
#5809=VERTEX_POINT('',#22319);
#5810=VERTEX_POINT('',#22321);
#5811=VERTEX_POINT('',#22323);
#5812=VERTEX_POINT('',#22325);
#5813=VERTEX_POINT('',#22327);
#5814=VERTEX_POINT('',#22330);
#5815=VERTEX_POINT('',#22334);
#5816=VERTEX_POINT('',#22336);
#5817=VERTEX_POINT('',#22340);
#5818=VERTEX_POINT('',#22341);
#5819=VERTEX_POINT('',#22346);
#5820=VERTEX_POINT('',#22347);
#5821=VERTEX_POINT('',#22352);
#5822=VERTEX_POINT('',#22353);
#5823=VERTEX_POINT('',#22358);
#5824=VERTEX_POINT('',#22359);
#5825=VERTEX_POINT('',#22364);
#5826=VERTEX_POINT('',#22369);
#5827=VERTEX_POINT('',#22376);
#5828=VERTEX_POINT('',#22382);
#5829=VERTEX_POINT('',#22383);
#5830=VERTEX_POINT('',#22385);
#5831=VERTEX_POINT('',#22387);
#5832=VERTEX_POINT('',#22389);
#5833=VERTEX_POINT('',#22391);
#5834=VERTEX_POINT('',#22393);
#5835=VERTEX_POINT('',#22395);
#5836=VERTEX_POINT('',#22399);
#5837=VERTEX_POINT('',#22403);
#5838=VERTEX_POINT('',#22407);
#5839=VERTEX_POINT('',#22411);
#5840=VERTEX_POINT('',#22415);
#5841=VERTEX_POINT('',#22419);
#5842=VERTEX_POINT('',#22423);
#5843=VERTEX_POINT('',#22427);
#5844=VERTEX_POINT('',#22431);
#5845=VERTEX_POINT('',#22435);
#5846=VERTEX_POINT('',#22439);
#5847=VERTEX_POINT('',#22443);
#5848=VERTEX_POINT('',#22447);
#5849=VERTEX_POINT('',#22451);
#5850=VERTEX_POINT('',#22452);
#5851=VERTEX_POINT('',#22454);
#5852=VERTEX_POINT('',#22456);
#5853=VERTEX_POINT('',#22459);
#5854=VERTEX_POINT('',#22461);
#5855=VERTEX_POINT('',#22463);
#5856=VERTEX_POINT('',#22465);
#5857=VERTEX_POINT('',#22467);
#5858=VERTEX_POINT('',#22469);
#5859=VERTEX_POINT('',#22484);
#5860=VERTEX_POINT('',#22486);
#5861=VERTEX_POINT('',#22490);
#5862=VERTEX_POINT('',#22494);
#5863=VERTEX_POINT('',#22498);
#5864=VERTEX_POINT('',#22502);
#5865=VERTEX_POINT('',#22513);
#5866=VERTEX_POINT('',#22517);
#5867=VERTEX_POINT('',#22521);
#5868=VERTEX_POINT('',#22524);
#5869=VERTEX_POINT('',#22526);
#5870=VERTEX_POINT('',#22528);
#5871=VERTEX_POINT('',#22530);
#5872=VERTEX_POINT('',#22532);
#5873=VERTEX_POINT('',#22534);
#5874=VERTEX_POINT('',#22549);
#5875=VERTEX_POINT('',#22551);
#5876=VERTEX_POINT('',#22555);
#5877=VERTEX_POINT('',#22559);
#5878=VERTEX_POINT('',#22563);
#5879=VERTEX_POINT('',#22564);
#5880=VERTEX_POINT('',#22569);
#5881=VERTEX_POINT('',#22570);
#5882=VERTEX_POINT('',#22575);
#5883=VERTEX_POINT('',#22576);
#5884=VERTEX_POINT('',#22581);
#5885=VERTEX_POINT('',#22590);
#5886=VERTEX_POINT('',#22591);
#5887=VERTEX_POINT('',#22593);
#5888=VERTEX_POINT('',#22595);
#5889=VERTEX_POINT('',#22597);
#5890=VERTEX_POINT('',#22599);
#5891=VERTEX_POINT('',#22601);
#5892=VERTEX_POINT('',#22603);
#5893=VERTEX_POINT('',#22614);
#5894=VERTEX_POINT('',#22618);
#5895=VERTEX_POINT('',#22622);
#7154=EDGE_CURVE('',#5780,#5780,#855,.T.);
#7155=EDGE_CURVE('',#5780,#5781,#3148,.T.);
#7156=EDGE_CURVE('',#5781,#5781,#856,.T.);
#7157=EDGE_CURVE('',#5782,#5783,#3149,.T.);
#7158=EDGE_CURVE('',#5782,#5784,#3150,.T.);
#7159=EDGE_CURVE('',#5785,#5784,#3151,.T.);
#7160=EDGE_CURVE('',#5783,#5785,#3152,.T.);
#7161=EDGE_CURVE('',#5786,#5786,#857,.T.);
#7162=EDGE_CURVE('',#5787,#5787,#858,.T.);
#7163=EDGE_CURVE('',#5788,#5788,#859,.T.);
#7164=EDGE_CURVE('',#5789,#5789,#860,.T.);
#7165=EDGE_CURVE('',#5790,#5790,#861,.T.);
#7166=EDGE_CURVE('',#5791,#5791,#862,.T.);
#7167=EDGE_CURVE('',#5791,#5781,#3153,.T.);
#7168=EDGE_CURVE('',#5786,#5792,#3154,.T.);
#7169=EDGE_CURVE('',#5792,#5792,#863,.T.);
#7170=EDGE_CURVE('',#5793,#5793,#864,.T.);
#7171=EDGE_CURVE('',#5793,#5792,#3155,.T.);
#7172=EDGE_CURVE('',#5790,#5794,#3156,.T.);
#7173=EDGE_CURVE('',#5794,#5794,#865,.T.);
#7174=EDGE_CURVE('',#5795,#5795,#866,.T.);
#7175=EDGE_CURVE('',#5795,#5794,#3157,.T.);
#7176=EDGE_CURVE('',#5787,#5796,#3158,.T.);
#7177=EDGE_CURVE('',#5796,#5796,#867,.T.);
#7178=EDGE_CURVE('',#5797,#5797,#868,.T.);
#7179=EDGE_CURVE('',#5797,#5796,#3159,.T.);
#7180=EDGE_CURVE('',#5789,#5798,#3160,.T.);
#7181=EDGE_CURVE('',#5798,#5798,#869,.T.);
#7182=EDGE_CURVE('',#5799,#5799,#870,.T.);
#7183=EDGE_CURVE('',#5799,#5798,#3161,.T.);
#7184=EDGE_CURVE('',#5788,#5800,#3162,.T.);
#7185=EDGE_CURVE('',#5800,#5800,#871,.T.);
#7186=EDGE_CURVE('',#5801,#5801,#872,.T.);
#7187=EDGE_CURVE('',#5801,#5800,#3163,.T.);
#7188=EDGE_CURVE('',#5802,#5802,#873,.T.);
#7189=EDGE_CURVE('',#5802,#5803,#3164,.T.);
#7190=EDGE_CURVE('',#5803,#5803,#874,.T.);
#7191=EDGE_CURVE('',#5804,#5805,#3165,.T.);
#7192=EDGE_CURVE('',#5804,#5806,#3166,.T.);
#7193=EDGE_CURVE('',#5807,#5806,#3167,.T.);
#7194=EDGE_CURVE('',#5805,#5807,#3168,.T.);
#7195=EDGE_CURVE('',#5808,#5808,#875,.T.);
#7196=EDGE_CURVE('',#5809,#5809,#876,.T.);
#7197=EDGE_CURVE('',#5810,#5810,#877,.T.);
#7198=EDGE_CURVE('',#5811,#5811,#878,.T.);
#7199=EDGE_CURVE('',#5812,#5812,#879,.T.);
#7200=EDGE_CURVE('',#5813,#5813,#880,.T.);
#7201=EDGE_CURVE('',#5814,#5814,#881,.T.);
#7202=EDGE_CURVE('',#5814,#5803,#3169,.T.);
#7203=EDGE_CURVE('',#5815,#5804,#3170,.T.);
#7204=EDGE_CURVE('',#5805,#5816,#3171,.T.);
#7205=EDGE_CURVE('',#5816,#5815,#3172,.T.);
#7206=EDGE_CURVE('',#5817,#5818,#3173,.T.);
#7207=EDGE_CURVE('',#5818,#5804,#882,.T.);
#7208=EDGE_CURVE('',#5815,#5817,#883,.T.);
#7209=EDGE_CURVE('',#5819,#5820,#3174,.T.);
#7210=EDGE_CURVE('',#5820,#5818,#3175,.T.);
#7211=EDGE_CURVE('',#5817,#5819,#3176,.T.);
#7212=EDGE_CURVE('',#5821,#5822,#3177,.T.);
#7213=EDGE_CURVE('',#5822,#5820,#884,.T.);
#7214=EDGE_CURVE('',#5819,#5821,#885,.T.);
#7215=EDGE_CURVE('',#5823,#5824,#3178,.T.);
#7216=EDGE_CURVE('',#5824,#5822,#3179,.T.);
#7217=EDGE_CURVE('',#5821,#5823,#3180,.T.);
#7218=EDGE_CURVE('',#5825,#5783,#3181,.T.);
#7219=EDGE_CURVE('',#5783,#5824,#886,.T.);
#7220=EDGE_CURVE('',#5823,#5825,#887,.T.);
#7221=EDGE_CURVE('',#5826,#5782,#3182,.T.);
#7222=EDGE_CURVE('',#5825,#5826,#3183,.T.);
#7223=EDGE_CURVE('',#5805,#5782,#888,.T.);
#7224=EDGE_CURVE('',#5826,#5816,#889,.T.);
#7225=EDGE_CURVE('',#5827,#5785,#890,.T.);
#7226=EDGE_CURVE('',#5824,#5827,#3184,.T.);
#7227=EDGE_CURVE('',#5784,#5807,#891,.T.);
#7228=EDGE_CURVE('',#5828,#5829,#3185,.T.);
#7229=EDGE_CURVE('',#5830,#5828,#892,.T.);
#7230=EDGE_CURVE('',#5831,#5830,#3186,.T.);
#7231=EDGE_CURVE('',#5832,#5831,#893,.T.);
#7232=EDGE_CURVE('',#5833,#5832,#3187,.T.);
#7233=EDGE_CURVE('',#5834,#5833,#894,.T.);
#7234=EDGE_CURVE('',#5835,#5834,#3188,.T.);
#7235=EDGE_CURVE('',#5829,#5835,#895,.T.);
#7236=EDGE_CURVE('',#5813,#5836,#3189,.T.);
#7237=EDGE_CURVE('',#5836,#5836,#896,.T.);
#7238=EDGE_CURVE('',#5837,#5837,#897,.T.);
#7239=EDGE_CURVE('',#5837,#5836,#3190,.T.);
#7240=EDGE_CURVE('',#5808,#5838,#3191,.T.);
#7241=EDGE_CURVE('',#5838,#5838,#898,.T.);
#7242=EDGE_CURVE('',#5839,#5839,#899,.T.);
#7243=EDGE_CURVE('',#5839,#5838,#3192,.T.);
#7244=EDGE_CURVE('',#5812,#5840,#3193,.T.);
#7245=EDGE_CURVE('',#5840,#5840,#900,.T.);
#7246=EDGE_CURVE('',#5841,#5841,#901,.T.);
#7247=EDGE_CURVE('',#5841,#5840,#3194,.T.);
#7248=EDGE_CURVE('',#5809,#5842,#3195,.T.);
#7249=EDGE_CURVE('',#5842,#5842,#902,.T.);
#7250=EDGE_CURVE('',#5843,#5843,#903,.T.);
#7251=EDGE_CURVE('',#5843,#5842,#3196,.T.);
#7252=EDGE_CURVE('',#5811,#5844,#3197,.T.);
#7253=EDGE_CURVE('',#5844,#5844,#904,.T.);
#7254=EDGE_CURVE('',#5845,#5845,#905,.T.);
#7255=EDGE_CURVE('',#5845,#5844,#3198,.T.);
#7256=EDGE_CURVE('',#5810,#5846,#3199,.T.);
#7257=EDGE_CURVE('',#5846,#5846,#906,.T.);
#7258=EDGE_CURVE('',#5847,#5847,#907,.T.);
#7259=EDGE_CURVE('',#5847,#5846,#3200,.T.);
#7260=EDGE_CURVE('',#5848,#5848,#908,.T.);
#7261=EDGE_CURVE('',#5848,#5837,#3201,.T.);
#7262=EDGE_CURVE('',#5849,#5850,#3202,.T.);
#7263=EDGE_CURVE('',#5849,#5851,#3203,.T.);
#7264=EDGE_CURVE('',#5852,#5851,#3204,.T.);
#7265=EDGE_CURVE('',#5850,#5852,#3205,.T.);
#7266=EDGE_CURVE('',#5853,#5853,#909,.T.);
#7267=EDGE_CURVE('',#5854,#5854,#910,.T.);
#7268=EDGE_CURVE('',#5855,#5855,#911,.T.);
#7269=EDGE_CURVE('',#5856,#5856,#912,.T.);
#7270=EDGE_CURVE('',#5857,#5857,#913,.T.);
#7271=EDGE_CURVE('',#5858,#5858,#914,.T.);
#7272=EDGE_CURVE('',#5853,#5814,#3206,.T.);
#7273=EDGE_CURVE('',#5858,#5839,#3207,.T.);
#7274=EDGE_CURVE('',#5854,#5841,#3208,.T.);
#7275=EDGE_CURVE('',#5857,#5843,#3209,.T.);
#7276=EDGE_CURVE('',#5855,#5845,#3210,.T.);
#7277=EDGE_CURVE('',#5856,#5847,#3211,.T.);
#7278=EDGE_CURVE('',#5829,#5859,#3212,.T.);
#7279=EDGE_CURVE('',#5859,#5860,#3213,.T.);
#7280=EDGE_CURVE('',#5860,#5828,#3214,.T.);
#7281=EDGE_CURVE('',#5835,#5861,#3215,.T.);
#7282=EDGE_CURVE('',#5861,#5859,#915,.T.);
#7283=EDGE_CURVE('',#5834,#5862,#3216,.T.);
#7284=EDGE_CURVE('',#5862,#5861,#3217,.T.);
#7285=EDGE_CURVE('',#5833,#5863,#3218,.T.);
#7286=EDGE_CURVE('',#5863,#5862,#916,.T.);
#7287=EDGE_CURVE('',#5832,#5864,#3219,.T.);
#7288=EDGE_CURVE('',#5864,#5863,#3220,.T.);
#7289=EDGE_CURVE('',#5831,#5850,#3221,.T.);
#7290=EDGE_CURVE('',#5850,#5864,#917,.T.);
#7291=EDGE_CURVE('',#5830,#5849,#3222,.T.);
#7292=EDGE_CURVE('',#5860,#5849,#918,.T.);
#7293=EDGE_CURVE('',#5865,#5852,#919,.T.);
#7294=EDGE_CURVE('',#5864,#5865,#3223,.T.);
#7295=EDGE_CURVE('',#5860,#5866,#3224,.T.);
#7296=EDGE_CURVE('',#5851,#5866,#920,.T.);
#7297=EDGE_CURVE('',#5859,#5867,#3225,.T.);
#7298=EDGE_CURVE('',#5866,#5867,#3226,.T.);
#7299=EDGE_CURVE('',#5868,#5868,#921,.T.);
#7300=EDGE_CURVE('',#5869,#5869,#922,.T.);
#7301=EDGE_CURVE('',#5870,#5870,#923,.T.);
#7302=EDGE_CURVE('',#5871,#5871,#924,.T.);
#7303=EDGE_CURVE('',#5872,#5872,#925,.T.);
#7304=EDGE_CURVE('',#5873,#5873,#926,.T.);
#7305=EDGE_CURVE('',#5868,#5801,#3227,.T.);
#7306=EDGE_CURVE('',#5873,#5799,#3228,.T.);
#7307=EDGE_CURVE('',#5869,#5797,#3229,.T.);
#7308=EDGE_CURVE('',#5872,#5795,#3230,.T.);
#7309=EDGE_CURVE('',#5870,#5793,#3231,.T.);
#7310=EDGE_CURVE('',#5871,#5791,#3232,.T.);
#7311=EDGE_CURVE('',#5851,#5874,#3233,.T.);
#7312=EDGE_CURVE('',#5874,#5875,#3234,.T.);
#7313=EDGE_CURVE('',#5875,#5852,#3235,.T.);
#7314=EDGE_CURVE('',#5866,#5876,#3236,.T.);
#7315=EDGE_CURVE('',#5876,#5874,#927,.T.);
#7316=EDGE_CURVE('',#5867,#5877,#3237,.T.);
#7317=EDGE_CURVE('',#5877,#5876,#3238,.T.);
#7318=EDGE_CURVE('',#5878,#5879,#3239,.T.);
#7319=EDGE_CURVE('',#5879,#5877,#928,.T.);
#7320=EDGE_CURVE('',#5867,#5878,#929,.T.);
#7321=EDGE_CURVE('',#5880,#5881,#3240,.T.);
#7322=EDGE_CURVE('',#5881,#5879,#3241,.T.);
#7323=EDGE_CURVE('',#5878,#5880,#3242,.T.);
#7324=EDGE_CURVE('',#5882,#5883,#3243,.T.);
#7325=EDGE_CURVE('',#5883,#5881,#930,.T.);
#7326=EDGE_CURVE('',#5880,#5882,#931,.T.);
#7327=EDGE_CURVE('',#5865,#5884,#3244,.T.);
#7328=EDGE_CURVE('',#5884,#5883,#3245,.T.);
#7329=EDGE_CURVE('',#5882,#5865,#3246,.T.);
#7330=EDGE_CURVE('',#5875,#5884,#932,.T.);
#7331=EDGE_CURVE('',#5861,#5878,#3247,.T.);
#7332=EDGE_CURVE('',#5885,#5886,#3248,.T.);
#7333=EDGE_CURVE('',#5887,#5885,#933,.T.);
#7334=EDGE_CURVE('',#5888,#5887,#3249,.T.);
#7335=EDGE_CURVE('',#5889,#5888,#934,.T.);
#7336=EDGE_CURVE('',#5890,#5889,#3250,.T.);
#7337=EDGE_CURVE('',#5891,#5890,#935,.T.);
#7338=EDGE_CURVE('',#5892,#5891,#3251,.T.);
#7339=EDGE_CURVE('',#5886,#5892,#936,.T.);
#7340=EDGE_CURVE('',#5784,#5885,#3252,.T.);
#7341=EDGE_CURVE('',#5886,#5785,#3253,.T.);
#7342=EDGE_CURVE('',#5807,#5887,#3254,.T.);
#7343=EDGE_CURVE('',#5806,#5888,#3255,.T.);
#7344=EDGE_CURVE('',#5893,#5889,#3256,.T.);
#7345=EDGE_CURVE('',#5806,#5893,#937,.T.);
#7346=EDGE_CURVE('',#5894,#5890,#3257,.T.);
#7347=EDGE_CURVE('',#5893,#5894,#3258,.T.);
#7348=EDGE_CURVE('',#5895,#5891,#3259,.T.);
#7349=EDGE_CURVE('',#5894,#5895,#938,.T.);
#7350=EDGE_CURVE('',#5827,#5892,#3260,.T.);
#7351=EDGE_CURVE('',#5895,#5827,#3261,.T.);
#7352=EDGE_CURVE('',#5818,#5893,#3262,.T.);
#7353=EDGE_CURVE('',#5822,#5895,#3263,.T.);
#7354=EDGE_CURVE('',#5820,#5894,#3264,.T.);
#7355=EDGE_CURVE('',#5863,#5882,#3265,.T.);
#7356=EDGE_CURVE('',#5862,#5880,#3266,.T.);
#9555=ORIENTED_EDGE('',*,*,#7154,.T.);
#9556=ORIENTED_EDGE('',*,*,#7155,.T.);
#9557=ORIENTED_EDGE('',*,*,#7156,.T.);
#9558=ORIENTED_EDGE('',*,*,#7155,.F.);
#9559=ORIENTED_EDGE('',*,*,#7157,.F.);
#9560=ORIENTED_EDGE('',*,*,#7158,.T.);
#9561=ORIENTED_EDGE('',*,*,#7159,.F.);
#9562=ORIENTED_EDGE('',*,*,#7160,.F.);
#9563=ORIENTED_EDGE('',*,*,#7161,.F.);
#9564=ORIENTED_EDGE('',*,*,#7162,.F.);
#9565=ORIENTED_EDGE('',*,*,#7163,.F.);
#9566=ORIENTED_EDGE('',*,*,#7164,.F.);
#9567=ORIENTED_EDGE('',*,*,#7165,.F.);
#9568=ORIENTED_EDGE('',*,*,#7154,.F.);
#9569=ORIENTED_EDGE('',*,*,#7166,.F.);
#9570=ORIENTED_EDGE('',*,*,#7167,.T.);
#9571=ORIENTED_EDGE('',*,*,#7156,.F.);
#9572=ORIENTED_EDGE('',*,*,#7167,.F.);
#9573=ORIENTED_EDGE('',*,*,#7161,.T.);
#9574=ORIENTED_EDGE('',*,*,#7168,.T.);
#9575=ORIENTED_EDGE('',*,*,#7169,.T.);
#9576=ORIENTED_EDGE('',*,*,#7168,.F.);
#9577=ORIENTED_EDGE('',*,*,#7170,.F.);
#9578=ORIENTED_EDGE('',*,*,#7171,.T.);
#9579=ORIENTED_EDGE('',*,*,#7169,.F.);
#9580=ORIENTED_EDGE('',*,*,#7171,.F.);
#9581=ORIENTED_EDGE('',*,*,#7165,.T.);
#9582=ORIENTED_EDGE('',*,*,#7172,.T.);
#9583=ORIENTED_EDGE('',*,*,#7173,.T.);
#9584=ORIENTED_EDGE('',*,*,#7172,.F.);
#9585=ORIENTED_EDGE('',*,*,#7174,.F.);
#9586=ORIENTED_EDGE('',*,*,#7175,.T.);
#9587=ORIENTED_EDGE('',*,*,#7173,.F.);
#9588=ORIENTED_EDGE('',*,*,#7175,.F.);
#9589=ORIENTED_EDGE('',*,*,#7162,.T.);
#9590=ORIENTED_EDGE('',*,*,#7176,.T.);
#9591=ORIENTED_EDGE('',*,*,#7177,.T.);
#9592=ORIENTED_EDGE('',*,*,#7176,.F.);
#9593=ORIENTED_EDGE('',*,*,#7178,.F.);
#9594=ORIENTED_EDGE('',*,*,#7179,.T.);
#9595=ORIENTED_EDGE('',*,*,#7177,.F.);
#9596=ORIENTED_EDGE('',*,*,#7179,.F.);
#9597=ORIENTED_EDGE('',*,*,#7164,.T.);
#9598=ORIENTED_EDGE('',*,*,#7180,.T.);
#9599=ORIENTED_EDGE('',*,*,#7181,.T.);
#9600=ORIENTED_EDGE('',*,*,#7180,.F.);
#9601=ORIENTED_EDGE('',*,*,#7182,.F.);
#9602=ORIENTED_EDGE('',*,*,#7183,.T.);
#9603=ORIENTED_EDGE('',*,*,#7181,.F.);
#9604=ORIENTED_EDGE('',*,*,#7183,.F.);
#9605=ORIENTED_EDGE('',*,*,#7163,.T.);
#9606=ORIENTED_EDGE('',*,*,#7184,.T.);
#9607=ORIENTED_EDGE('',*,*,#7185,.T.);
#9608=ORIENTED_EDGE('',*,*,#7184,.F.);
#9609=ORIENTED_EDGE('',*,*,#7186,.F.);
#9610=ORIENTED_EDGE('',*,*,#7187,.T.);
#9611=ORIENTED_EDGE('',*,*,#7185,.F.);
#9612=ORIENTED_EDGE('',*,*,#7187,.F.);
#9613=ORIENTED_EDGE('',*,*,#7188,.T.);
#9614=ORIENTED_EDGE('',*,*,#7189,.T.);
#9615=ORIENTED_EDGE('',*,*,#7190,.T.);
#9616=ORIENTED_EDGE('',*,*,#7189,.F.);
#9617=ORIENTED_EDGE('',*,*,#7191,.F.);
#9618=ORIENTED_EDGE('',*,*,#7192,.T.);
#9619=ORIENTED_EDGE('',*,*,#7193,.F.);
#9620=ORIENTED_EDGE('',*,*,#7194,.F.);
#9621=ORIENTED_EDGE('',*,*,#7195,.F.);
#9622=ORIENTED_EDGE('',*,*,#7196,.F.);
#9623=ORIENTED_EDGE('',*,*,#7197,.F.);
#9624=ORIENTED_EDGE('',*,*,#7198,.F.);
#9625=ORIENTED_EDGE('',*,*,#7199,.F.);
#9626=ORIENTED_EDGE('',*,*,#7200,.F.);
#9627=ORIENTED_EDGE('',*,*,#7188,.F.);
#9628=ORIENTED_EDGE('',*,*,#7201,.F.);
#9629=ORIENTED_EDGE('',*,*,#7202,.T.);
#9630=ORIENTED_EDGE('',*,*,#7190,.F.);
#9631=ORIENTED_EDGE('',*,*,#7202,.F.);
#9632=ORIENTED_EDGE('',*,*,#7203,.T.);
#9633=ORIENTED_EDGE('',*,*,#7191,.T.);
#9634=ORIENTED_EDGE('',*,*,#7204,.T.);
#9635=ORIENTED_EDGE('',*,*,#7205,.T.);
#9636=ORIENTED_EDGE('',*,*,#7206,.T.);
#9637=ORIENTED_EDGE('',*,*,#7207,.T.);
#9638=ORIENTED_EDGE('',*,*,#7203,.F.);
#9639=ORIENTED_EDGE('',*,*,#7208,.T.);
#9640=ORIENTED_EDGE('',*,*,#7209,.T.);
#9641=ORIENTED_EDGE('',*,*,#7210,.T.);
#9642=ORIENTED_EDGE('',*,*,#7206,.F.);
#9643=ORIENTED_EDGE('',*,*,#7211,.T.);
#9644=ORIENTED_EDGE('',*,*,#7212,.T.);
#9645=ORIENTED_EDGE('',*,*,#7213,.T.);
#9646=ORIENTED_EDGE('',*,*,#7209,.F.);
#9647=ORIENTED_EDGE('',*,*,#7214,.T.);
#9648=ORIENTED_EDGE('',*,*,#7215,.T.);
#9649=ORIENTED_EDGE('',*,*,#7216,.T.);
#9650=ORIENTED_EDGE('',*,*,#7212,.F.);
#9651=ORIENTED_EDGE('',*,*,#7217,.T.);
#9652=ORIENTED_EDGE('',*,*,#7218,.T.);
#9653=ORIENTED_EDGE('',*,*,#7219,.T.);
#9654=ORIENTED_EDGE('',*,*,#7215,.F.);
#9655=ORIENTED_EDGE('',*,*,#7220,.T.);
#9656=ORIENTED_EDGE('',*,*,#7221,.T.);
#9657=ORIENTED_EDGE('',*,*,#7157,.T.);
#9658=ORIENTED_EDGE('',*,*,#7218,.F.);
#9659=ORIENTED_EDGE('',*,*,#7222,.T.);
#9660=ORIENTED_EDGE('',*,*,#7204,.F.);
#9661=ORIENTED_EDGE('',*,*,#7223,.T.);
#9662=ORIENTED_EDGE('',*,*,#7221,.F.);
#9663=ORIENTED_EDGE('',*,*,#7224,.T.);
#9664=ORIENTED_EDGE('',*,*,#7219,.F.);
#9665=ORIENTED_EDGE('',*,*,#7160,.T.);
#9666=ORIENTED_EDGE('',*,*,#7225,.F.);
#9667=ORIENTED_EDGE('',*,*,#7226,.F.);
#9668=ORIENTED_EDGE('',*,*,#7223,.F.);
#9669=ORIENTED_EDGE('',*,*,#7194,.T.);
#9670=ORIENTED_EDGE('',*,*,#7227,.F.);
#9671=ORIENTED_EDGE('',*,*,#7158,.F.);
#9672=ORIENTED_EDGE('',*,*,#7228,.F.);
#9673=ORIENTED_EDGE('',*,*,#7229,.F.);
#9674=ORIENTED_EDGE('',*,*,#7230,.F.);
#9675=ORIENTED_EDGE('',*,*,#7231,.F.);
#9676=ORIENTED_EDGE('',*,*,#7232,.F.);
#9677=ORIENTED_EDGE('',*,*,#7233,.F.);
#9678=ORIENTED_EDGE('',*,*,#7234,.F.);
#9679=ORIENTED_EDGE('',*,*,#7235,.F.);
#9680=ORIENTED_EDGE('',*,*,#7205,.F.);
#9681=ORIENTED_EDGE('',*,*,#7224,.F.);
#9682=ORIENTED_EDGE('',*,*,#7222,.F.);
#9683=ORIENTED_EDGE('',*,*,#7220,.F.);
#9684=ORIENTED_EDGE('',*,*,#7217,.F.);
#9685=ORIENTED_EDGE('',*,*,#7214,.F.);
#9686=ORIENTED_EDGE('',*,*,#7211,.F.);
#9687=ORIENTED_EDGE('',*,*,#7208,.F.);
#9688=ORIENTED_EDGE('',*,*,#7200,.T.);
#9689=ORIENTED_EDGE('',*,*,#7236,.T.);
#9690=ORIENTED_EDGE('',*,*,#7237,.T.);
#9691=ORIENTED_EDGE('',*,*,#7236,.F.);
#9692=ORIENTED_EDGE('',*,*,#7238,.F.);
#9693=ORIENTED_EDGE('',*,*,#7239,.T.);
#9694=ORIENTED_EDGE('',*,*,#7237,.F.);
#9695=ORIENTED_EDGE('',*,*,#7239,.F.);
#9696=ORIENTED_EDGE('',*,*,#7195,.T.);
#9697=ORIENTED_EDGE('',*,*,#7240,.T.);
#9698=ORIENTED_EDGE('',*,*,#7241,.T.);
#9699=ORIENTED_EDGE('',*,*,#7240,.F.);
#9700=ORIENTED_EDGE('',*,*,#7242,.F.);
#9701=ORIENTED_EDGE('',*,*,#7243,.T.);
#9702=ORIENTED_EDGE('',*,*,#7241,.F.);
#9703=ORIENTED_EDGE('',*,*,#7243,.F.);
#9704=ORIENTED_EDGE('',*,*,#7199,.T.);
#9705=ORIENTED_EDGE('',*,*,#7244,.T.);
#9706=ORIENTED_EDGE('',*,*,#7245,.T.);
#9707=ORIENTED_EDGE('',*,*,#7244,.F.);
#9708=ORIENTED_EDGE('',*,*,#7246,.F.);
#9709=ORIENTED_EDGE('',*,*,#7247,.T.);
#9710=ORIENTED_EDGE('',*,*,#7245,.F.);
#9711=ORIENTED_EDGE('',*,*,#7247,.F.);
#9712=ORIENTED_EDGE('',*,*,#7196,.T.);
#9713=ORIENTED_EDGE('',*,*,#7248,.T.);
#9714=ORIENTED_EDGE('',*,*,#7249,.T.);
#9715=ORIENTED_EDGE('',*,*,#7248,.F.);
#9716=ORIENTED_EDGE('',*,*,#7250,.F.);
#9717=ORIENTED_EDGE('',*,*,#7251,.T.);
#9718=ORIENTED_EDGE('',*,*,#7249,.F.);
#9719=ORIENTED_EDGE('',*,*,#7251,.F.);
#9720=ORIENTED_EDGE('',*,*,#7198,.T.);
#9721=ORIENTED_EDGE('',*,*,#7252,.T.);
#9722=ORIENTED_EDGE('',*,*,#7253,.T.);
#9723=ORIENTED_EDGE('',*,*,#7252,.F.);
#9724=ORIENTED_EDGE('',*,*,#7254,.F.);
#9725=ORIENTED_EDGE('',*,*,#7255,.T.);
#9726=ORIENTED_EDGE('',*,*,#7253,.F.);
#9727=ORIENTED_EDGE('',*,*,#7255,.F.);
#9728=ORIENTED_EDGE('',*,*,#7197,.T.);
#9729=ORIENTED_EDGE('',*,*,#7256,.T.);
#9730=ORIENTED_EDGE('',*,*,#7257,.T.);
#9731=ORIENTED_EDGE('',*,*,#7256,.F.);
#9732=ORIENTED_EDGE('',*,*,#7258,.F.);
#9733=ORIENTED_EDGE('',*,*,#7259,.T.);
#9734=ORIENTED_EDGE('',*,*,#7257,.F.);
#9735=ORIENTED_EDGE('',*,*,#7259,.F.);
#9736=ORIENTED_EDGE('',*,*,#7260,.T.);
#9737=ORIENTED_EDGE('',*,*,#7261,.T.);
#9738=ORIENTED_EDGE('',*,*,#7238,.T.);
#9739=ORIENTED_EDGE('',*,*,#7261,.F.);
#9740=ORIENTED_EDGE('',*,*,#7262,.F.);
#9741=ORIENTED_EDGE('',*,*,#7263,.T.);
#9742=ORIENTED_EDGE('',*,*,#7264,.F.);
#9743=ORIENTED_EDGE('',*,*,#7265,.F.);
#9744=ORIENTED_EDGE('',*,*,#7266,.F.);
#9745=ORIENTED_EDGE('',*,*,#7267,.F.);
#9746=ORIENTED_EDGE('',*,*,#7268,.F.);
#9747=ORIENTED_EDGE('',*,*,#7269,.F.);
#9748=ORIENTED_EDGE('',*,*,#7270,.F.);
#9749=ORIENTED_EDGE('',*,*,#7271,.F.);
#9750=ORIENTED_EDGE('',*,*,#7260,.F.);
#9751=ORIENTED_EDGE('',*,*,#7266,.T.);
#9752=ORIENTED_EDGE('',*,*,#7272,.T.);
#9753=ORIENTED_EDGE('',*,*,#7201,.T.);
#9754=ORIENTED_EDGE('',*,*,#7272,.F.);
#9755=ORIENTED_EDGE('',*,*,#7271,.T.);
#9756=ORIENTED_EDGE('',*,*,#7273,.T.);
#9757=ORIENTED_EDGE('',*,*,#7242,.T.);
#9758=ORIENTED_EDGE('',*,*,#7273,.F.);
#9759=ORIENTED_EDGE('',*,*,#7267,.T.);
#9760=ORIENTED_EDGE('',*,*,#7274,.T.);
#9761=ORIENTED_EDGE('',*,*,#7246,.T.);
#9762=ORIENTED_EDGE('',*,*,#7274,.F.);
#9763=ORIENTED_EDGE('',*,*,#7270,.T.);
#9764=ORIENTED_EDGE('',*,*,#7275,.T.);
#9765=ORIENTED_EDGE('',*,*,#7250,.T.);
#9766=ORIENTED_EDGE('',*,*,#7275,.F.);
#9767=ORIENTED_EDGE('',*,*,#7268,.T.);
#9768=ORIENTED_EDGE('',*,*,#7276,.T.);
#9769=ORIENTED_EDGE('',*,*,#7254,.T.);
#9770=ORIENTED_EDGE('',*,*,#7276,.F.);
#9771=ORIENTED_EDGE('',*,*,#7269,.T.);
#9772=ORIENTED_EDGE('',*,*,#7277,.T.);
#9773=ORIENTED_EDGE('',*,*,#7258,.T.);
#9774=ORIENTED_EDGE('',*,*,#7277,.F.);
#9775=ORIENTED_EDGE('',*,*,#7278,.T.);
#9776=ORIENTED_EDGE('',*,*,#7279,.T.);
#9777=ORIENTED_EDGE('',*,*,#7280,.T.);
#9778=ORIENTED_EDGE('',*,*,#7228,.T.);
#9779=ORIENTED_EDGE('',*,*,#7281,.T.);
#9780=ORIENTED_EDGE('',*,*,#7282,.T.);
#9781=ORIENTED_EDGE('',*,*,#7278,.F.);
#9782=ORIENTED_EDGE('',*,*,#7235,.T.);
#9783=ORIENTED_EDGE('',*,*,#7283,.T.);
#9784=ORIENTED_EDGE('',*,*,#7284,.T.);
#9785=ORIENTED_EDGE('',*,*,#7281,.F.);
#9786=ORIENTED_EDGE('',*,*,#7234,.T.);
#9787=ORIENTED_EDGE('',*,*,#7285,.T.);
#9788=ORIENTED_EDGE('',*,*,#7286,.T.);
#9789=ORIENTED_EDGE('',*,*,#7283,.F.);
#9790=ORIENTED_EDGE('',*,*,#7233,.T.);
#9791=ORIENTED_EDGE('',*,*,#7287,.T.);
#9792=ORIENTED_EDGE('',*,*,#7288,.T.);
#9793=ORIENTED_EDGE('',*,*,#7285,.F.);
#9794=ORIENTED_EDGE('',*,*,#7232,.T.);
#9795=ORIENTED_EDGE('',*,*,#7289,.T.);
#9796=ORIENTED_EDGE('',*,*,#7290,.T.);
#9797=ORIENTED_EDGE('',*,*,#7287,.F.);
#9798=ORIENTED_EDGE('',*,*,#7231,.T.);
#9799=ORIENTED_EDGE('',*,*,#7291,.T.);
#9800=ORIENTED_EDGE('',*,*,#7262,.T.);
#9801=ORIENTED_EDGE('',*,*,#7289,.F.);
#9802=ORIENTED_EDGE('',*,*,#7230,.T.);
#9803=ORIENTED_EDGE('',*,*,#7280,.F.);
#9804=ORIENTED_EDGE('',*,*,#7292,.T.);
#9805=ORIENTED_EDGE('',*,*,#7291,.F.);
#9806=ORIENTED_EDGE('',*,*,#7229,.T.);
#9807=ORIENTED_EDGE('',*,*,#7290,.F.);
#9808=ORIENTED_EDGE('',*,*,#7265,.T.);
#9809=ORIENTED_EDGE('',*,*,#7293,.F.);
#9810=ORIENTED_EDGE('',*,*,#7294,.F.);
#9811=ORIENTED_EDGE('',*,*,#7292,.F.);
#9812=ORIENTED_EDGE('',*,*,#7295,.T.);
#9813=ORIENTED_EDGE('',*,*,#7296,.F.);
#9814=ORIENTED_EDGE('',*,*,#7263,.F.);
#9815=ORIENTED_EDGE('',*,*,#7279,.F.);
#9816=ORIENTED_EDGE('',*,*,#7297,.T.);
#9817=ORIENTED_EDGE('',*,*,#7298,.F.);
#9818=ORIENTED_EDGE('',*,*,#7295,.F.);
#9819=ORIENTED_EDGE('',*,*,#7299,.F.);
#9820=ORIENTED_EDGE('',*,*,#7300,.F.);
#9821=ORIENTED_EDGE('',*,*,#7301,.F.);
#9822=ORIENTED_EDGE('',*,*,#7302,.F.);
#9823=ORIENTED_EDGE('',*,*,#7303,.F.);
#9824=ORIENTED_EDGE('',*,*,#7304,.F.);
#9825=ORIENTED_EDGE('',*,*,#7299,.T.);
#9826=ORIENTED_EDGE('',*,*,#7305,.T.);
#9827=ORIENTED_EDGE('',*,*,#7186,.T.);
#9828=ORIENTED_EDGE('',*,*,#7305,.F.);
#9829=ORIENTED_EDGE('',*,*,#7304,.T.);
#9830=ORIENTED_EDGE('',*,*,#7306,.T.);
#9831=ORIENTED_EDGE('',*,*,#7182,.T.);
#9832=ORIENTED_EDGE('',*,*,#7306,.F.);
#9833=ORIENTED_EDGE('',*,*,#7300,.T.);
#9834=ORIENTED_EDGE('',*,*,#7307,.T.);
#9835=ORIENTED_EDGE('',*,*,#7178,.T.);
#9836=ORIENTED_EDGE('',*,*,#7307,.F.);
#9837=ORIENTED_EDGE('',*,*,#7303,.T.);
#9838=ORIENTED_EDGE('',*,*,#7308,.T.);
#9839=ORIENTED_EDGE('',*,*,#7174,.T.);
#9840=ORIENTED_EDGE('',*,*,#7308,.F.);
#9841=ORIENTED_EDGE('',*,*,#7301,.T.);
#9842=ORIENTED_EDGE('',*,*,#7309,.T.);
#9843=ORIENTED_EDGE('',*,*,#7170,.T.);
#9844=ORIENTED_EDGE('',*,*,#7309,.F.);
#9845=ORIENTED_EDGE('',*,*,#7302,.T.);
#9846=ORIENTED_EDGE('',*,*,#7310,.T.);
#9847=ORIENTED_EDGE('',*,*,#7166,.T.);
#9848=ORIENTED_EDGE('',*,*,#7310,.F.);
#9849=ORIENTED_EDGE('',*,*,#7311,.T.);
#9850=ORIENTED_EDGE('',*,*,#7312,.T.);
#9851=ORIENTED_EDGE('',*,*,#7313,.T.);
#9852=ORIENTED_EDGE('',*,*,#7264,.T.);
#9853=ORIENTED_EDGE('',*,*,#7314,.T.);
#9854=ORIENTED_EDGE('',*,*,#7315,.T.);
#9855=ORIENTED_EDGE('',*,*,#7311,.F.);
#9856=ORIENTED_EDGE('',*,*,#7296,.T.);
#9857=ORIENTED_EDGE('',*,*,#7316,.T.);
#9858=ORIENTED_EDGE('',*,*,#7317,.T.);
#9859=ORIENTED_EDGE('',*,*,#7314,.F.);
#9860=ORIENTED_EDGE('',*,*,#7298,.T.);
#9861=ORIENTED_EDGE('',*,*,#7318,.T.);
#9862=ORIENTED_EDGE('',*,*,#7319,.T.);
#9863=ORIENTED_EDGE('',*,*,#7316,.F.);
#9864=ORIENTED_EDGE('',*,*,#7320,.T.);
#9865=ORIENTED_EDGE('',*,*,#7321,.T.);
#9866=ORIENTED_EDGE('',*,*,#7322,.T.);
#9867=ORIENTED_EDGE('',*,*,#7318,.F.);
#9868=ORIENTED_EDGE('',*,*,#7323,.T.);
#9869=ORIENTED_EDGE('',*,*,#7324,.T.);
#9870=ORIENTED_EDGE('',*,*,#7325,.T.);
#9871=ORIENTED_EDGE('',*,*,#7321,.F.);
#9872=ORIENTED_EDGE('',*,*,#7326,.T.);
#9873=ORIENTED_EDGE('',*,*,#7327,.T.);
#9874=ORIENTED_EDGE('',*,*,#7328,.T.);
#9875=ORIENTED_EDGE('',*,*,#7324,.F.);
#9876=ORIENTED_EDGE('',*,*,#7329,.T.);
#9877=ORIENTED_EDGE('',*,*,#7313,.F.);
#9878=ORIENTED_EDGE('',*,*,#7330,.T.);
#9879=ORIENTED_EDGE('',*,*,#7327,.F.);
#9880=ORIENTED_EDGE('',*,*,#7293,.T.);
#9881=ORIENTED_EDGE('',*,*,#7282,.F.);
#9882=ORIENTED_EDGE('',*,*,#7331,.T.);
#9883=ORIENTED_EDGE('',*,*,#7320,.F.);
#9884=ORIENTED_EDGE('',*,*,#7297,.F.);
#9885=ORIENTED_EDGE('',*,*,#7312,.F.);
#9886=ORIENTED_EDGE('',*,*,#7315,.F.);
#9887=ORIENTED_EDGE('',*,*,#7317,.F.);
#9888=ORIENTED_EDGE('',*,*,#7319,.F.);
#9889=ORIENTED_EDGE('',*,*,#7322,.F.);
#9890=ORIENTED_EDGE('',*,*,#7325,.F.);
#9891=ORIENTED_EDGE('',*,*,#7328,.F.);
#9892=ORIENTED_EDGE('',*,*,#7330,.F.);
#9893=ORIENTED_EDGE('',*,*,#7332,.F.);
#9894=ORIENTED_EDGE('',*,*,#7333,.F.);
#9895=ORIENTED_EDGE('',*,*,#7334,.F.);
#9896=ORIENTED_EDGE('',*,*,#7335,.F.);
#9897=ORIENTED_EDGE('',*,*,#7336,.F.);
#9898=ORIENTED_EDGE('',*,*,#7337,.F.);
#9899=ORIENTED_EDGE('',*,*,#7338,.F.);
#9900=ORIENTED_EDGE('',*,*,#7339,.F.);
#9901=ORIENTED_EDGE('',*,*,#7340,.T.);
#9902=ORIENTED_EDGE('',*,*,#7332,.T.);
#9903=ORIENTED_EDGE('',*,*,#7341,.T.);
#9904=ORIENTED_EDGE('',*,*,#7159,.T.);
#9905=ORIENTED_EDGE('',*,*,#7342,.T.);
#9906=ORIENTED_EDGE('',*,*,#7333,.T.);
#9907=ORIENTED_EDGE('',*,*,#7340,.F.);
#9908=ORIENTED_EDGE('',*,*,#7227,.T.);
#9909=ORIENTED_EDGE('',*,*,#7343,.T.);
#9910=ORIENTED_EDGE('',*,*,#7334,.T.);
#9911=ORIENTED_EDGE('',*,*,#7342,.F.);
#9912=ORIENTED_EDGE('',*,*,#7193,.T.);
#9913=ORIENTED_EDGE('',*,*,#7344,.T.);
#9914=ORIENTED_EDGE('',*,*,#7335,.T.);
#9915=ORIENTED_EDGE('',*,*,#7343,.F.);
#9916=ORIENTED_EDGE('',*,*,#7345,.T.);
#9917=ORIENTED_EDGE('',*,*,#7346,.T.);
#9918=ORIENTED_EDGE('',*,*,#7336,.T.);
#9919=ORIENTED_EDGE('',*,*,#7344,.F.);
#9920=ORIENTED_EDGE('',*,*,#7347,.T.);
#9921=ORIENTED_EDGE('',*,*,#7348,.T.);
#9922=ORIENTED_EDGE('',*,*,#7337,.T.);
#9923=ORIENTED_EDGE('',*,*,#7346,.F.);
#9924=ORIENTED_EDGE('',*,*,#7349,.T.);
#9925=ORIENTED_EDGE('',*,*,#7350,.T.);
#9926=ORIENTED_EDGE('',*,*,#7338,.T.);
#9927=ORIENTED_EDGE('',*,*,#7348,.F.);
#9928=ORIENTED_EDGE('',*,*,#7351,.T.);
#9929=ORIENTED_EDGE('',*,*,#7341,.F.);
#9930=ORIENTED_EDGE('',*,*,#7339,.T.);
#9931=ORIENTED_EDGE('',*,*,#7350,.F.);
#9932=ORIENTED_EDGE('',*,*,#7225,.T.);
#9933=ORIENTED_EDGE('',*,*,#7207,.F.);
#9934=ORIENTED_EDGE('',*,*,#7352,.T.);
#9935=ORIENTED_EDGE('',*,*,#7345,.F.);
#9936=ORIENTED_EDGE('',*,*,#7192,.F.);
#9937=ORIENTED_EDGE('',*,*,#7216,.F.);
#9938=ORIENTED_EDGE('',*,*,#7226,.T.);
#9939=ORIENTED_EDGE('',*,*,#7351,.F.);
#9940=ORIENTED_EDGE('',*,*,#7353,.F.);
#9941=ORIENTED_EDGE('',*,*,#7213,.F.);
#9942=ORIENTED_EDGE('',*,*,#7353,.T.);
#9943=ORIENTED_EDGE('',*,*,#7349,.F.);
#9944=ORIENTED_EDGE('',*,*,#7354,.F.);
#9945=ORIENTED_EDGE('',*,*,#7210,.F.);
#9946=ORIENTED_EDGE('',*,*,#7354,.T.);
#9947=ORIENTED_EDGE('',*,*,#7347,.F.);
#9948=ORIENTED_EDGE('',*,*,#7352,.F.);
#9949=ORIENTED_EDGE('',*,*,#7288,.F.);
#9950=ORIENTED_EDGE('',*,*,#7294,.T.);
#9951=ORIENTED_EDGE('',*,*,#7329,.F.);
#9952=ORIENTED_EDGE('',*,*,#7355,.F.);
#9953=ORIENTED_EDGE('',*,*,#7286,.F.);
#9954=ORIENTED_EDGE('',*,*,#7355,.T.);
#9955=ORIENTED_EDGE('',*,*,#7326,.F.);
#9956=ORIENTED_EDGE('',*,*,#7356,.F.);
#9957=ORIENTED_EDGE('',*,*,#7284,.F.);
#9958=ORIENTED_EDGE('',*,*,#7356,.T.);
#9959=ORIENTED_EDGE('',*,*,#7323,.F.);
#9960=ORIENTED_EDGE('',*,*,#7331,.F.);
#12673=PLANE('',#14208);
#12674=PLANE('',#14239);
#12675=PLANE('',#14248);
#12676=PLANE('',#14252);
#12677=PLANE('',#14256);
#12678=PLANE('',#14260);
#12679=PLANE('',#14268);
#12680=PLANE('',#14299);
#12681=PLANE('',#14312);
#12682=PLANE('',#14315);
#12683=PLANE('',#14318);
#12684=PLANE('',#14321);
#12685=PLANE('',#14328);
#12686=PLANE('',#14341);
#12687=PLANE('',#14344);
#12688=PLANE('',#14348);
#12689=PLANE('',#14352);
#12690=PLANE('',#14356);
#12691=PLANE('',#14361);
#12692=PLANE('',#14363);
#12693=PLANE('',#14366);
#12694=PLANE('',#14369);
#12695=PLANE('',#14372);
#12696=PLANE('',#14374);
#12697=PLANE('',#14375);
#12698=PLANE('',#14377);
#13189=ADVANCED_FACE('',(#1426),#1135,.F.);
#13190=ADVANCED_FACE('',(#1427,#599,#600,#601,#602,#603,#604),#12673,.T.);
#13191=ADVANCED_FACE('',(#1428),#685,.F.);
#13192=ADVANCED_FACE('',(#1429),#1136,.F.);
#13193=ADVANCED_FACE('',(#1430),#686,.F.);
#13194=ADVANCED_FACE('',(#1431),#1137,.F.);
#13195=ADVANCED_FACE('',(#1432),#687,.F.);
#13196=ADVANCED_FACE('',(#1433),#1138,.F.);
#13197=ADVANCED_FACE('',(#1434),#688,.F.);
#13198=ADVANCED_FACE('',(#1435),#1139,.F.);
#13199=ADVANCED_FACE('',(#1436),#689,.F.);
#13200=ADVANCED_FACE('',(#1437),#1140,.F.);
#13201=ADVANCED_FACE('',(#1438),#690,.F.);
#13202=ADVANCED_FACE('',(#1439),#1141,.F.);
#13203=ADVANCED_FACE('',(#1440,#605,#606,#607,#608,#609,#610,#611),#12674,
 .T.);
#13204=ADVANCED_FACE('',(#1441),#691,.F.);
#13205=ADVANCED_FACE('',(#1442),#12675,.T.);
#13206=ADVANCED_FACE('',(#1443),#1142,.F.);
#13207=ADVANCED_FACE('',(#1444),#12676,.T.);
#13208=ADVANCED_FACE('',(#1445),#1143,.F.);
#13209=ADVANCED_FACE('',(#1446),#12677,.T.);
#13210=ADVANCED_FACE('',(#1447),#1144,.F.);
#13211=ADVANCED_FACE('',(#1448),#12678,.T.);
#13212=ADVANCED_FACE('',(#1449),#1145,.F.);
#13213=ADVANCED_FACE('',(#1450),#692,.F.);
#13214=ADVANCED_FACE('',(#1451),#693,.F.);
#13215=ADVANCED_FACE('',(#1452,#612),#12679,.F.);
#13216=ADVANCED_FACE('',(#1453),#1146,.F.);
#13217=ADVANCED_FACE('',(#1454),#694,.F.);
#13218=ADVANCED_FACE('',(#1455),#1147,.F.);
#13219=ADVANCED_FACE('',(#1456),#695,.F.);
#13220=ADVANCED_FACE('',(#1457),#1148,.F.);
#13221=ADVANCED_FACE('',(#1458),#696,.F.);
#13222=ADVANCED_FACE('',(#1459),#1149,.F.);
#13223=ADVANCED_FACE('',(#1460),#697,.F.);
#13224=ADVANCED_FACE('',(#1461),#1150,.F.);
#13225=ADVANCED_FACE('',(#1462),#698,.F.);
#13226=ADVANCED_FACE('',(#1463),#1151,.F.);
#13227=ADVANCED_FACE('',(#1464),#699,.F.);
#13228=ADVANCED_FACE('',(#1465),#1152,.F.);
#13229=ADVANCED_FACE('',(#1466,#613,#614,#615,#616,#617,#618,#619),#12680,
 .T.);
#13230=ADVANCED_FACE('',(#1467),#1153,.F.);
#13231=ADVANCED_FACE('',(#1468),#1154,.F.);
#13232=ADVANCED_FACE('',(#1469),#1155,.F.);
#13233=ADVANCED_FACE('',(#1470),#1156,.F.);
#13234=ADVANCED_FACE('',(#1471),#1157,.F.);
#13235=ADVANCED_FACE('',(#1472),#1158,.F.);
#13236=ADVANCED_FACE('',(#1473),#12681,.T.);
#13237=ADVANCED_FACE('',(#1474),#1159,.T.);
#13238=ADVANCED_FACE('',(#1475),#12682,.T.);
#13239=ADVANCED_FACE('',(#1476),#1160,.T.);
#13240=ADVANCED_FACE('',(#1477),#12683,.T.);
#13241=ADVANCED_FACE('',(#1478),#1161,.T.);
#13242=ADVANCED_FACE('',(#1479),#12684,.T.);
#13243=ADVANCED_FACE('',(#1480),#1162,.T.);
#13244=ADVANCED_FACE('',(#1481),#700,.T.);
#13245=ADVANCED_FACE('',(#1482),#701,.T.);
#13246=ADVANCED_FACE('',(#1483,#620,#621,#622,#623,#624,#625),#12685,.T.);
#13247=ADVANCED_FACE('',(#1484),#1163,.F.);
#13248=ADVANCED_FACE('',(#1485),#1164,.F.);
#13249=ADVANCED_FACE('',(#1486),#1165,.F.);
#13250=ADVANCED_FACE('',(#1487),#1166,.F.);
#13251=ADVANCED_FACE('',(#1488),#1167,.F.);
#13252=ADVANCED_FACE('',(#1489),#1168,.F.);
#13253=ADVANCED_FACE('',(#1490),#12686,.T.);
#13254=ADVANCED_FACE('',(#1491),#1169,.T.);
#13255=ADVANCED_FACE('',(#1492),#12687,.T.);
#13256=ADVANCED_FACE('',(#1493),#1170,.T.);
#13257=ADVANCED_FACE('',(#1494),#12688,.T.);
#13258=ADVANCED_FACE('',(#1495),#1171,.T.);
#13259=ADVANCED_FACE('',(#1496),#12689,.T.);
#13260=ADVANCED_FACE('',(#1497),#1172,.T.);
#13261=ADVANCED_FACE('',(#1498),#702,.T.);
#13262=ADVANCED_FACE('',(#1499,#626),#12690,.T.);
#13263=ADVANCED_FACE('',(#1500),#12691,.T.);
#13264=ADVANCED_FACE('',(#1501),#1173,.F.);
#13265=ADVANCED_FACE('',(#1502),#12692,.T.);
#13266=ADVANCED_FACE('',(#1503),#1174,.F.);
#13267=ADVANCED_FACE('',(#1504),#12693,.T.);
#13268=ADVANCED_FACE('',(#1505),#1175,.F.);
#13269=ADVANCED_FACE('',(#1506),#12694,.T.);
#13270=ADVANCED_FACE('',(#1507),#1176,.F.);
#13271=ADVANCED_FACE('',(#1508),#703,.F.);
#13272=ADVANCED_FACE('',(#1509),#12695,.T.);
#13273=ADVANCED_FACE('',(#1510),#704,.F.);
#13274=ADVANCED_FACE('',(#1511),#12696,.T.);
#13275=ADVANCED_FACE('',(#1512),#12697,.T.);
#13276=ADVANCED_FACE('',(#1513),#705,.T.);
#13277=ADVANCED_FACE('',(#1514),#12698,.T.);
#13808=CLOSED_SHELL('',(#13189,#13190,#13191,#13192,#13193,#13194,#13195,
#13196,#13197,#13198,#13199,#13200,#13201,#13202,#13203,#13204,#13205,#13206,
#13207,#13208,#13209,#13210,#13211,#13212,#13213,#13214,#13215,#13216,#13217,
#13218,#13219,#13220,#13221,#13222,#13223,#13224,#13225,#13226,#13227,#13228,
#13229,#13230,#13231,#13232,#13233,#13234,#13235,#13236,#13237,#13238,#13239,
#13240,#13241,#13242,#13243,#13244,#13245,#13246,#13247,#13248,#13249,#13250,
#13251,#13252,#13253,#13254,#13255,#13256,#13257,#13258,#13259,#13260,#13261,
#13262,#13263,#13264,#13265,#13266,#13267,#13268,#13269,#13270,#13271,#13272,
#13273,#13274,#13275,#13276,#13277));
#14204=AXIS2_PLACEMENT_3D('',#22232,#15718,#15719);
#14205=AXIS2_PLACEMENT_3D('',#22233,#15720,#15721);
#14206=AXIS2_PLACEMENT_3D('',#22235,#15722,#15723);
#14207=AXIS2_PLACEMENT_3D('',#22238,#15725,#15726);
#14208=AXIS2_PLACEMENT_3D('',#22239,#15727,#15728);
#14209=AXIS2_PLACEMENT_3D('',#22249,#15733,#15734);
#14210=AXIS2_PLACEMENT_3D('',#22251,#15735,#15736);
#14211=AXIS2_PLACEMENT_3D('',#22253,#15737,#15738);
#14212=AXIS2_PLACEMENT_3D('',#22255,#15739,#15740);
#14213=AXIS2_PLACEMENT_3D('',#22257,#15741,#15742);
#14214=AXIS2_PLACEMENT_3D('',#22258,#15743,#15744);
#14215=AXIS2_PLACEMENT_3D('',#22260,#15745,#15746);
#14216=AXIS2_PLACEMENT_3D('',#22262,#15748,#15749);
#14217=AXIS2_PLACEMENT_3D('',#22265,#15751,#15752);
#14218=AXIS2_PLACEMENT_3D('',#22266,#15753,#15754);
#14219=AXIS2_PLACEMENT_3D('',#22268,#15755,#15756);
#14220=AXIS2_PLACEMENT_3D('',#22270,#15758,#15759);
#14221=AXIS2_PLACEMENT_3D('',#22273,#15761,#15762);
#14222=AXIS2_PLACEMENT_3D('',#22274,#15763,#15764);
#14223=AXIS2_PLACEMENT_3D('',#22276,#15765,#15766);
#14224=AXIS2_PLACEMENT_3D('',#22278,#15768,#15769);
#14225=AXIS2_PLACEMENT_3D('',#22281,#15771,#15772);
#14226=AXIS2_PLACEMENT_3D('',#22282,#15773,#15774);
#14227=AXIS2_PLACEMENT_3D('',#22284,#15775,#15776);
#14228=AXIS2_PLACEMENT_3D('',#22286,#15778,#15779);
#14229=AXIS2_PLACEMENT_3D('',#22289,#15781,#15782);
#14230=AXIS2_PLACEMENT_3D('',#22290,#15783,#15784);
#14231=AXIS2_PLACEMENT_3D('',#22292,#15785,#15786);
#14232=AXIS2_PLACEMENT_3D('',#22294,#15788,#15789);
#14233=AXIS2_PLACEMENT_3D('',#22297,#15791,#15792);
#14234=AXIS2_PLACEMENT_3D('',#22298,#15793,#15794);
#14235=AXIS2_PLACEMENT_3D('',#22300,#15795,#15796);
#14236=AXIS2_PLACEMENT_3D('',#22302,#15798,#15799);
#14237=AXIS2_PLACEMENT_3D('',#22304,#15800,#15801);
#14238=AXIS2_PLACEMENT_3D('',#22307,#15803,#15804);
#14239=AXIS2_PLACEMENT_3D('',#22308,#15805,#15806);
#14240=AXIS2_PLACEMENT_3D('',#22318,#15811,#15812);
#14241=AXIS2_PLACEMENT_3D('',#22320,#15813,#15814);
#14242=AXIS2_PLACEMENT_3D('',#22322,#15815,#15816);
#14243=AXIS2_PLACEMENT_3D('',#22324,#15817,#15818);
#14244=AXIS2_PLACEMENT_3D('',#22326,#15819,#15820);
#14245=AXIS2_PLACEMENT_3D('',#22328,#15821,#15822);
#14246=AXIS2_PLACEMENT_3D('',#22329,#15823,#15824);
#14247=AXIS2_PLACEMENT_3D('',#22331,#15825,#15826);
#14248=AXIS2_PLACEMENT_3D('',#22333,#15828,#15829);
#14249=AXIS2_PLACEMENT_3D('',#22339,#15833,#15834);
#14250=AXIS2_PLACEMENT_3D('',#22343,#15836,#15837);
#14251=AXIS2_PLACEMENT_3D('',#22344,#15838,#15839);
#14252=AXIS2_PLACEMENT_3D('',#22345,#15840,#15841);
#14253=AXIS2_PLACEMENT_3D('',#22351,#15845,#15846);
#14254=AXIS2_PLACEMENT_3D('',#22355,#15848,#15849);
#14255=AXIS2_PLACEMENT_3D('',#22356,#15850,#15851);
#14256=AXIS2_PLACEMENT_3D('',#22357,#15852,#15853);
#14257=AXIS2_PLACEMENT_3D('',#22363,#15857,#15858);
#14258=AXIS2_PLACEMENT_3D('',#22366,#15860,#15861);
#14259=AXIS2_PLACEMENT_3D('',#22367,#15862,#15863);
#14260=AXIS2_PLACEMENT_3D('',#22368,#15864,#15865);
#14261=AXIS2_PLACEMENT_3D('',#22372,#15868,#15869);
#14262=AXIS2_PLACEMENT_3D('',#22373,#15870,#15871);
#14263=AXIS2_PLACEMENT_3D('',#22374,#15872,#15873);
#14264=AXIS2_PLACEMENT_3D('',#22375,#15874,#15875);
#14265=AXIS2_PLACEMENT_3D('',#22377,#15876,#15877);
#14266=AXIS2_PLACEMENT_3D('',#22379,#15879,#15880);
#14267=AXIS2_PLACEMENT_3D('',#22380,#15881,#15882);
#14268=AXIS2_PLACEMENT_3D('',#22381,#15883,#15884);
#14269=AXIS2_PLACEMENT_3D('',#22386,#15886,#15887);
#14270=AXIS2_PLACEMENT_3D('',#22390,#15889,#15890);
#14271=AXIS2_PLACEMENT_3D('',#22394,#15892,#15893);
#14272=AXIS2_PLACEMENT_3D('',#22397,#15895,#15896);
#14273=AXIS2_PLACEMENT_3D('',#22398,#15897,#15898);
#14274=AXIS2_PLACEMENT_3D('',#22401,#15900,#15901);
#14275=AXIS2_PLACEMENT_3D('',#22402,#15902,#15903);
#14276=AXIS2_PLACEMENT_3D('',#22404,#15904,#15905);
#14277=AXIS2_PLACEMENT_3D('',#22406,#15907,#15908);
#14278=AXIS2_PLACEMENT_3D('',#22409,#15910,#15911);
#14279=AXIS2_PLACEMENT_3D('',#22410,#15912,#15913);
#14280=AXIS2_PLACEMENT_3D('',#22412,#15914,#15915);
#14281=AXIS2_PLACEMENT_3D('',#22414,#15917,#15918);
#14282=AXIS2_PLACEMENT_3D('',#22417,#15920,#15921);
#14283=AXIS2_PLACEMENT_3D('',#22418,#15922,#15923);
#14284=AXIS2_PLACEMENT_3D('',#22420,#15924,#15925);
#14285=AXIS2_PLACEMENT_3D('',#22422,#15927,#15928);
#14286=AXIS2_PLACEMENT_3D('',#22425,#15930,#15931);
#14287=AXIS2_PLACEMENT_3D('',#22426,#15932,#15933);
#14288=AXIS2_PLACEMENT_3D('',#22428,#15934,#15935);
#14289=AXIS2_PLACEMENT_3D('',#22430,#15937,#15938);
#14290=AXIS2_PLACEMENT_3D('',#22433,#15940,#15941);
#14291=AXIS2_PLACEMENT_3D('',#22434,#15942,#15943);
#14292=AXIS2_PLACEMENT_3D('',#22436,#15944,#15945);
#14293=AXIS2_PLACEMENT_3D('',#22438,#15947,#15948);
#14294=AXIS2_PLACEMENT_3D('',#22441,#15950,#15951);
#14295=AXIS2_PLACEMENT_3D('',#22442,#15952,#15953);
#14296=AXIS2_PLACEMENT_3D('',#22444,#15954,#15955);
#14297=AXIS2_PLACEMENT_3D('',#22446,#15957,#15958);
#14298=AXIS2_PLACEMENT_3D('',#22448,#15959,#15960);
#14299=AXIS2_PLACEMENT_3D('',#22450,#15962,#15963);
#14300=AXIS2_PLACEMENT_3D('',#22460,#15968,#15969);
#14301=AXIS2_PLACEMENT_3D('',#22462,#15970,#15971);
#14302=AXIS2_PLACEMENT_3D('',#22464,#15972,#15973);
#14303=AXIS2_PLACEMENT_3D('',#22466,#15974,#15975);
#14304=AXIS2_PLACEMENT_3D('',#22468,#15976,#15977);
#14305=AXIS2_PLACEMENT_3D('',#22470,#15978,#15979);
#14306=AXIS2_PLACEMENT_3D('',#22471,#15980,#15981);
#14307=AXIS2_PLACEMENT_3D('',#22473,#15983,#15984);
#14308=AXIS2_PLACEMENT_3D('',#22475,#15986,#15987);
#14309=AXIS2_PLACEMENT_3D('',#22477,#15989,#15990);
#14310=AXIS2_PLACEMENT_3D('',#22479,#15992,#15993);
#14311=AXIS2_PLACEMENT_3D('',#22481,#15995,#15996);
#14312=AXIS2_PLACEMENT_3D('',#22483,#15998,#15999);
#14313=AXIS2_PLACEMENT_3D('',#22489,#16003,#16004);
#14314=AXIS2_PLACEMENT_3D('',#22492,#16006,#16007);
#14315=AXIS2_PLACEMENT_3D('',#22493,#16008,#16009);
#14316=AXIS2_PLACEMENT_3D('',#22497,#16012,#16013);
#14317=AXIS2_PLACEMENT_3D('',#22500,#16015,#16016);
#14318=AXIS2_PLACEMENT_3D('',#22501,#16017,#16018);
#14319=AXIS2_PLACEMENT_3D('',#22505,#16021,#16022);
#14320=AXIS2_PLACEMENT_3D('',#22507,#16024,#16025);
#14321=AXIS2_PLACEMENT_3D('',#22508,#16026,#16027);
#14322=AXIS2_PLACEMENT_3D('',#22510,#16029,#16030);
#14323=AXIS2_PLACEMENT_3D('',#22511,#16031,#16032);
#14324=AXIS2_PLACEMENT_3D('',#22512,#16033,#16034);
#14325=AXIS2_PLACEMENT_3D('',#22514,#16035,#16036);
#14326=AXIS2_PLACEMENT_3D('',#22516,#16038,#16039);
#14327=AXIS2_PLACEMENT_3D('',#22519,#16041,#16042);
#14328=AXIS2_PLACEMENT_3D('',#22520,#16043,#16044);
#14329=AXIS2_PLACEMENT_3D('',#22525,#16047,#16048);
#14330=AXIS2_PLACEMENT_3D('',#22527,#16049,#16050);
#14331=AXIS2_PLACEMENT_3D('',#22529,#16051,#16052);
#14332=AXIS2_PLACEMENT_3D('',#22531,#16053,#16054);
#14333=AXIS2_PLACEMENT_3D('',#22533,#16055,#16056);
#14334=AXIS2_PLACEMENT_3D('',#22535,#16057,#16058);
#14335=AXIS2_PLACEMENT_3D('',#22536,#16059,#16060);
#14336=AXIS2_PLACEMENT_3D('',#22538,#16062,#16063);
#14337=AXIS2_PLACEMENT_3D('',#22540,#16065,#16066);
#14338=AXIS2_PLACEMENT_3D('',#22542,#16068,#16069);
#14339=AXIS2_PLACEMENT_3D('',#22544,#16071,#16072);
#14340=AXIS2_PLACEMENT_3D('',#22546,#16074,#16075);
#14341=AXIS2_PLACEMENT_3D('',#22548,#16077,#16078);
#14342=AXIS2_PLACEMENT_3D('',#22554,#16082,#16083);
#14343=AXIS2_PLACEMENT_3D('',#22557,#16085,#16086);
#14344=AXIS2_PLACEMENT_3D('',#22558,#16087,#16088);
#14345=AXIS2_PLACEMENT_3D('',#22562,#16091,#16092);
#14346=AXIS2_PLACEMENT_3D('',#22566,#16094,#16095);
#14347=AXIS2_PLACEMENT_3D('',#22567,#16096,#16097);
#14348=AXIS2_PLACEMENT_3D('',#22568,#16098,#16099);
#14349=AXIS2_PLACEMENT_3D('',#22574,#16103,#16104);
#14350=AXIS2_PLACEMENT_3D('',#22578,#16106,#16107);
#14351=AXIS2_PLACEMENT_3D('',#22579,#16108,#16109);
#14352=AXIS2_PLACEMENT_3D('',#22580,#16110,#16111);
#14353=AXIS2_PLACEMENT_3D('',#22585,#16115,#16116);
#14354=AXIS2_PLACEMENT_3D('',#22586,#16117,#16118);
#14355=AXIS2_PLACEMENT_3D('',#22587,#16119,#16120);
#14356=AXIS2_PLACEMENT_3D('',#22589,#16122,#16123);
#14357=AXIS2_PLACEMENT_3D('',#22594,#16125,#16126);
#14358=AXIS2_PLACEMENT_3D('',#22598,#16128,#16129);
#14359=AXIS2_PLACEMENT_3D('',#22602,#16131,#16132);
#14360=AXIS2_PLACEMENT_3D('',#22605,#16134,#16135);
#14361=AXIS2_PLACEMENT_3D('',#22606,#16136,#16137);
#14362=AXIS2_PLACEMENT_3D('',#22609,#16140,#16141);
#14363=AXIS2_PLACEMENT_3D('',#22611,#16143,#16144);
#14364=AXIS2_PLACEMENT_3D('',#22613,#16146,#16147);
#14365=AXIS2_PLACEMENT_3D('',#22616,#16149,#16150);
#14366=AXIS2_PLACEMENT_3D('',#22617,#16151,#16152);
#14367=AXIS2_PLACEMENT_3D('',#22621,#16155,#16156);
#14368=AXIS2_PLACEMENT_3D('',#22624,#16158,#16159);
#14369=AXIS2_PLACEMENT_3D('',#22625,#16160,#16161);
#14370=AXIS2_PLACEMENT_3D('',#22628,#16164,#16165);
#14371=AXIS2_PLACEMENT_3D('',#22629,#16166,#16167);
#14372=AXIS2_PLACEMENT_3D('',#22631,#16169,#16170);
#14373=AXIS2_PLACEMENT_3D('',#22633,#16172,#16173);
#14374=AXIS2_PLACEMENT_3D('',#22635,#16175,#16176);
#14375=AXIS2_PLACEMENT_3D('',#22636,#16177,#16178);
#14376=AXIS2_PLACEMENT_3D('',#22638,#16180,#16181);
#14377=AXIS2_PLACEMENT_3D('',#22640,#16183,#16184);
#15718=DIRECTION('axis',(0.,0.,1.));
#15719=DIRECTION('refdir',(1.,0.,0.));
#15720=DIRECTION('center_axis',(0.,0.,1.));
#15721=DIRECTION('ref_axis',(1.,0.,0.));
#15722=DIRECTION('center_axis',(0.,0.,1.));
#15723=DIRECTION('ref_axis',(1.,0.,0.));
#15724=DIRECTION('',(0.707106781186547,8.65956056235493E-17,-0.707106781186547));
#15725=DIRECTION('center_axis',(0.,0.,-1.));
#15726=DIRECTION('ref_axis',(1.,0.,0.));
#15727=DIRECTION('center_axis',(0.,0.,1.));
#15728=DIRECTION('ref_axis',(0.,-1.,0.));
#15729=DIRECTION('',(0.,1.,0.));
#15730=DIRECTION('',(1.,0.,0.));
#15731=DIRECTION('',(0.,-1.,0.));
#15732=DIRECTION('',(1.,0.,0.));
#15733=DIRECTION('center_axis',(0.,0.,1.));
#15734=DIRECTION('ref_axis',(1.,0.,0.));
#15735=DIRECTION('center_axis',(0.,0.,1.));
#15736=DIRECTION('ref_axis',(1.,0.,0.));
#15737=DIRECTION('center_axis',(0.,0.,1.));
#15738=DIRECTION('ref_axis',(1.,0.,0.));
#15739=DIRECTION('center_axis',(0.,0.,1.));
#15740=DIRECTION('ref_axis',(1.,0.,0.));
#15741=DIRECTION('center_axis',(0.,0.,1.));
#15742=DIRECTION('ref_axis',(1.,0.,0.));
#15743=DIRECTION('center_axis',(0.,0.,1.));
#15744=DIRECTION('ref_axis',(1.,0.,0.));
#15745=DIRECTION('center_axis',(0.,0.,1.));
#15746=DIRECTION('ref_axis',(1.,0.,0.));
#15747=DIRECTION('',(0.,0.,1.));
#15748=DIRECTION('center_axis',(0.,0.,1.));
#15749=DIRECTION('ref_axis',(1.,0.,0.));
#15750=DIRECTION('',(0.707106781186549,8.65956056235495E-17,-0.707106781186546));
#15751=DIRECTION('center_axis',(0.,0.,-1.));
#15752=DIRECTION('ref_axis',(1.,0.,0.));
#15753=DIRECTION('center_axis',(0.,0.,1.));
#15754=DIRECTION('ref_axis',(1.,0.,0.));
#15755=DIRECTION('center_axis',(0.,0.,1.));
#15756=DIRECTION('ref_axis',(1.,0.,0.));
#15757=DIRECTION('',(0.,0.,1.));
#15758=DIRECTION('center_axis',(0.,0.,1.));
#15759=DIRECTION('ref_axis',(1.,0.,0.));
#15760=DIRECTION('',(0.707106781186549,8.65956056235495E-17,-0.707106781186546));
#15761=DIRECTION('center_axis',(0.,0.,-1.));
#15762=DIRECTION('ref_axis',(1.,0.,0.));
#15763=DIRECTION('center_axis',(0.,0.,1.));
#15764=DIRECTION('ref_axis',(1.,0.,0.));
#15765=DIRECTION('center_axis',(0.,0.,1.));
#15766=DIRECTION('ref_axis',(1.,0.,0.));
#15767=DIRECTION('',(0.,0.,1.));
#15768=DIRECTION('center_axis',(0.,0.,1.));
#15769=DIRECTION('ref_axis',(1.,0.,0.));
#15770=DIRECTION('',(0.707106781186548,8.65956056235493E-17,-0.707106781186548));
#15771=DIRECTION('center_axis',(0.,0.,-1.));
#15772=DIRECTION('ref_axis',(1.,0.,0.));
#15773=DIRECTION('center_axis',(0.,0.,1.));
#15774=DIRECTION('ref_axis',(1.,0.,0.));
#15775=DIRECTION('center_axis',(0.,0.,1.));
#15776=DIRECTION('ref_axis',(1.,0.,0.));
#15777=DIRECTION('',(0.,0.,1.));
#15778=DIRECTION('center_axis',(0.,0.,1.));
#15779=DIRECTION('ref_axis',(1.,0.,0.));
#15780=DIRECTION('',(0.707106781186547,8.65956056235493E-17,-0.707106781186547));
#15781=DIRECTION('center_axis',(0.,0.,-1.));
#15782=DIRECTION('ref_axis',(1.,0.,0.));
#15783=DIRECTION('center_axis',(0.,0.,1.));
#15784=DIRECTION('ref_axis',(1.,0.,0.));
#15785=DIRECTION('center_axis',(0.,0.,1.));
#15786=DIRECTION('ref_axis',(1.,0.,0.));
#15787=DIRECTION('',(0.,0.,1.));
#15788=DIRECTION('center_axis',(0.,0.,1.));
#15789=DIRECTION('ref_axis',(1.,0.,0.));
#15790=DIRECTION('',(0.707106781186547,8.65956056235493E-17,-0.707106781186547));
#15791=DIRECTION('center_axis',(0.,0.,-1.));
#15792=DIRECTION('ref_axis',(1.,0.,0.));
#15793=DIRECTION('center_axis',(0.,0.,1.));
#15794=DIRECTION('ref_axis',(1.,0.,0.));
#15795=DIRECTION('center_axis',(0.,0.,1.));
#15796=DIRECTION('ref_axis',(1.,0.,0.));
#15797=DIRECTION('',(0.,0.,1.));
#15798=DIRECTION('center_axis',(0.,1.,0.));
#15799=DIRECTION('ref_axis',(1.,0.,0.));
#15800=DIRECTION('center_axis',(0.,1.,0.));
#15801=DIRECTION('ref_axis',(1.,0.,0.));
#15802=DIRECTION('',(0.707106781186546,-0.707106781186549,-8.65956056235491E-17));
#15803=DIRECTION('center_axis',(0.,-1.,0.));
#15804=DIRECTION('ref_axis',(1.,0.,0.));
#15805=DIRECTION('center_axis',(0.,1.,0.));
#15806=DIRECTION('ref_axis',(0.,0.,1.));
#15807=DIRECTION('',(0.,0.,-1.));
#15808=DIRECTION('',(1.,0.,0.));
#15809=DIRECTION('',(0.,0.,1.));
#15810=DIRECTION('',(1.,0.,0.));
#15811=DIRECTION('center_axis',(0.,1.,0.));
#15812=DIRECTION('ref_axis',(1.,0.,0.));
#15813=DIRECTION('center_axis',(0.,1.,0.));
#15814=DIRECTION('ref_axis',(1.,0.,0.));
#15815=DIRECTION('center_axis',(0.,1.,0.));
#15816=DIRECTION('ref_axis',(1.,0.,0.));
#15817=DIRECTION('center_axis',(0.,1.,0.));
#15818=DIRECTION('ref_axis',(1.,0.,0.));
#15819=DIRECTION('center_axis',(0.,1.,0.));
#15820=DIRECTION('ref_axis',(1.,0.,0.));
#15821=DIRECTION('center_axis',(0.,1.,0.));
#15822=DIRECTION('ref_axis',(1.,0.,0.));
#15823=DIRECTION('center_axis',(0.,1.,0.));
#15824=DIRECTION('ref_axis',(1.,0.,0.));
#15825=DIRECTION('center_axis',(0.,1.,0.));
#15826=DIRECTION('ref_axis',(1.,0.,0.));
#15827=DIRECTION('',(0.,1.,0.));
#15828=DIRECTION('center_axis',(-0.707106781186548,0.707106781186548,0.));
#15829=DIRECTION('ref_axis',(0.,0.,1.));
#15830=DIRECTION('',(0.707106781186548,0.707106781186548,-3.14018491736756E-15));
#15831=DIRECTION('',(-0.707106781186548,-0.707106781186548,0.));
#15832=DIRECTION('',(0.,0.,1.));
#15833=DIRECTION('center_axis',(-1.,0.,0.));
#15834=DIRECTION('ref_axis',(0.,1.79429983777803E-15,1.));
#15835=DIRECTION('',(0.707106781186548,0.,-0.707106781186548));
#15836=DIRECTION('center_axis',(1.,0.,0.));
#15837=DIRECTION('ref_axis',(0.,1.79429983777803E-15,1.));
#15838=DIRECTION('center_axis',(-1.,0.,0.));
#15839=DIRECTION('ref_axis',(0.,1.79429983777803E-15,1.));
#15840=DIRECTION('center_axis',(-0.707106781186548,0.,-0.707106781186548));
#15841=DIRECTION('ref_axis',(-0.707106781186548,0.,0.707106781186548));
#15842=DIRECTION('',(0.707106781186541,0.,-0.707106781186554));
#15843=DIRECTION('',(0.,-1.,0.));
#15844=DIRECTION('',(0.,1.,0.));
#15845=DIRECTION('center_axis',(-1.,0.,0.));
#15846=DIRECTION('ref_axis',(0.,1.,1.79429983777804E-15));
#15847=DIRECTION('',(0.707106781186548,-0.707106781186548,0.));
#15848=DIRECTION('center_axis',(1.,0.,0.));
#15849=DIRECTION('ref_axis',(0.,1.,1.79429983777804E-15));
#15850=DIRECTION('center_axis',(-1.,0.,0.));
#15851=DIRECTION('ref_axis',(0.,1.,1.79429983777804E-15));
#15852=DIRECTION('center_axis',(-0.707106781186548,-0.707106781186548,0.));
#15853=DIRECTION('ref_axis',(0.,0.,1.));
#15854=DIRECTION('',(0.707106781186554,-0.707106781186541,3.14018491736759E-15));
#15855=DIRECTION('',(0.,0.,1.));
#15856=DIRECTION('',(0.,0.,-1.));
#15857=DIRECTION('center_axis',(-1.,0.,0.));
#15858=DIRECTION('ref_axis',(0.,-7.17719935111212E-15,-1.));
#15859=DIRECTION('',(0.707106781186548,0.,0.707106781186548));
#15860=DIRECTION('center_axis',(1.,0.,0.));
#15861=DIRECTION('ref_axis',(0.,-7.17719935111212E-15,-1.));
#15862=DIRECTION('center_axis',(-1.,0.,0.));
#15863=DIRECTION('ref_axis',(0.,-7.17719935111212E-15,-1.));
#15864=DIRECTION('center_axis',(-0.707106781186548,0.,0.707106781186548));
#15865=DIRECTION('ref_axis',(0.707106781186548,0.,0.707106781186548));
#15866=DIRECTION('',(0.707106781186548,-3.14018491736756E-15,0.707106781186548));
#15867=DIRECTION('',(0.,-1.,0.));
#15868=DIRECTION('center_axis',(-1.,0.,0.));
#15869=DIRECTION('ref_axis',(0.,-1.,0.));
#15870=DIRECTION('center_axis',(1.,0.,0.));
#15871=DIRECTION('ref_axis',(0.,-1.,0.));
#15872=DIRECTION('center_axis',(-1.,0.,0.));
#15873=DIRECTION('ref_axis',(0.,-1.,0.));
#15874=DIRECTION('center_axis',(1.,0.,0.));
#15875=DIRECTION('ref_axis',(0.,-7.17719935111212E-15,-1.));
#15876=DIRECTION('center_axis',(-1.,0.,0.));
#15877=DIRECTION('ref_axis',(0.,-7.17719935111212E-15,-1.));
#15878=DIRECTION('',(1.,0.,0.));
#15879=DIRECTION('center_axis',(1.,0.,0.));
#15880=DIRECTION('ref_axis',(0.,-1.,0.));
#15881=DIRECTION('center_axis',(-1.,0.,0.));
#15882=DIRECTION('ref_axis',(0.,-1.,0.));
#15883=DIRECTION('center_axis',(1.,0.,0.));
#15884=DIRECTION('ref_axis',(0.,0.,-1.));
#15885=DIRECTION('',(0.,1.,0.));
#15886=DIRECTION('center_axis',(1.,0.,0.));
#15887=DIRECTION('ref_axis',(0.,-1.,-1.48029736616687E-15));
#15888=DIRECTION('',(0.,0.,-1.));
#15889=DIRECTION('center_axis',(1.,0.,0.));
#15890=DIRECTION('ref_axis',(0.,-1.85037170770859E-15,1.));
#15891=DIRECTION('',(0.,-1.,0.));
#15892=DIRECTION('center_axis',(1.,0.,0.));
#15893=DIRECTION('ref_axis',(0.,1.,2.22044604925031E-15));
#15894=DIRECTION('',(0.,0.,1.));
#15895=DIRECTION('center_axis',(1.,0.,0.));
#15896=DIRECTION('ref_axis',(0.,2.96059473233374E-15,-1.));
#15897=DIRECTION('center_axis',(0.,1.,0.));
#15898=DIRECTION('ref_axis',(1.,0.,0.));
#15899=DIRECTION('',(0.707106781186546,-0.707106781186549,-8.65956056235492E-17));
#15900=DIRECTION('center_axis',(0.,-1.,0.));
#15901=DIRECTION('ref_axis',(1.,0.,0.));
#15902=DIRECTION('center_axis',(0.,1.,0.));
#15903=DIRECTION('ref_axis',(1.,0.,0.));
#15904=DIRECTION('center_axis',(0.,1.,0.));
#15905=DIRECTION('ref_axis',(1.,0.,0.));
#15906=DIRECTION('',(0.,1.,0.));
#15907=DIRECTION('center_axis',(0.,1.,0.));
#15908=DIRECTION('ref_axis',(1.,0.,0.));
#15909=DIRECTION('',(0.707106781186546,-0.707106781186549,-8.65956056235491E-17));
#15910=DIRECTION('center_axis',(0.,-1.,0.));
#15911=DIRECTION('ref_axis',(1.,0.,0.));
#15912=DIRECTION('center_axis',(0.,1.,0.));
#15913=DIRECTION('ref_axis',(1.,0.,0.));
#15914=DIRECTION('center_axis',(0.,1.,0.));
#15915=DIRECTION('ref_axis',(1.,0.,0.));
#15916=DIRECTION('',(0.,1.,0.));
#15917=DIRECTION('center_axis',(0.,1.,0.));
#15918=DIRECTION('ref_axis',(1.,0.,0.));
#15919=DIRECTION('',(0.707106781186546,-0.707106781186549,-8.65956056235491E-17));
#15920=DIRECTION('center_axis',(0.,-1.,0.));
#15921=DIRECTION('ref_axis',(1.,0.,0.));
#15922=DIRECTION('center_axis',(0.,1.,0.));
#15923=DIRECTION('ref_axis',(1.,0.,0.));
#15924=DIRECTION('center_axis',(0.,1.,0.));
#15925=DIRECTION('ref_axis',(1.,0.,0.));
#15926=DIRECTION('',(0.,1.,0.));
#15927=DIRECTION('center_axis',(0.,1.,0.));
#15928=DIRECTION('ref_axis',(1.,0.,0.));
#15929=DIRECTION('',(0.707106781186547,-0.707106781186547,-8.65956056235493E-17));
#15930=DIRECTION('center_axis',(0.,-1.,0.));
#15931=DIRECTION('ref_axis',(1.,0.,0.));
#15932=DIRECTION('center_axis',(0.,1.,0.));
#15933=DIRECTION('ref_axis',(1.,0.,0.));
#15934=DIRECTION('center_axis',(0.,1.,0.));
#15935=DIRECTION('ref_axis',(1.,0.,0.));
#15936=DIRECTION('',(0.,1.,0.));
#15937=DIRECTION('center_axis',(0.,1.,0.));
#15938=DIRECTION('ref_axis',(1.,0.,0.));
#15939=DIRECTION('',(0.707106781186547,-0.707106781186547,-8.65956056235493E-17));
#15940=DIRECTION('center_axis',(0.,-1.,0.));
#15941=DIRECTION('ref_axis',(1.,0.,0.));
#15942=DIRECTION('center_axis',(0.,1.,0.));
#15943=DIRECTION('ref_axis',(1.,0.,0.));
#15944=DIRECTION('center_axis',(0.,1.,0.));
#15945=DIRECTION('ref_axis',(1.,0.,0.));
#15946=DIRECTION('',(0.,1.,0.));
#15947=DIRECTION('center_axis',(0.,1.,0.));
#15948=DIRECTION('ref_axis',(1.,0.,0.));
#15949=DIRECTION('',(0.707106781186546,-0.707106781186549,-8.65956056235491E-17));
#15950=DIRECTION('center_axis',(0.,-1.,0.));
#15951=DIRECTION('ref_axis',(1.,0.,0.));
#15952=DIRECTION('center_axis',(0.,1.,0.));
#15953=DIRECTION('ref_axis',(1.,0.,0.));
#15954=DIRECTION('center_axis',(0.,1.,0.));
#15955=DIRECTION('ref_axis',(1.,0.,0.));
#15956=DIRECTION('',(0.,1.,0.));
#15957=DIRECTION('center_axis',(0.,-1.,0.));
#15958=DIRECTION('ref_axis',(1.,0.,0.));
#15959=DIRECTION('center_axis',(0.,-1.,0.));
#15960=DIRECTION('ref_axis',(1.,0.,0.));
#15961=DIRECTION('',(0.707106781186546,0.707106781186549,8.65956056235492E-17));
#15962=DIRECTION('center_axis',(0.,-1.,0.));
#15963=DIRECTION('ref_axis',(0.,0.,-1.));
#15964=DIRECTION('',(0.,0.,1.));
#15965=DIRECTION('',(1.,0.,0.));
#15966=DIRECTION('',(0.,0.,-1.));
#15967=DIRECTION('',(1.,0.,0.));
#15968=DIRECTION('center_axis',(0.,-1.,0.));
#15969=DIRECTION('ref_axis',(1.,0.,0.));
#15970=DIRECTION('center_axis',(0.,-1.,0.));
#15971=DIRECTION('ref_axis',(1.,0.,0.));
#15972=DIRECTION('center_axis',(0.,-1.,0.));
#15973=DIRECTION('ref_axis',(1.,0.,0.));
#15974=DIRECTION('center_axis',(0.,-1.,0.));
#15975=DIRECTION('ref_axis',(1.,0.,0.));
#15976=DIRECTION('center_axis',(0.,-1.,0.));
#15977=DIRECTION('ref_axis',(1.,0.,0.));
#15978=DIRECTION('center_axis',(0.,-1.,0.));
#15979=DIRECTION('ref_axis',(1.,0.,0.));
#15980=DIRECTION('center_axis',(0.,-1.,0.));
#15981=DIRECTION('ref_axis',(1.,0.,0.));
#15982=DIRECTION('',(0.707106781186546,0.707106781186549,8.65956056235491E-17));
#15983=DIRECTION('center_axis',(0.,-1.,0.));
#15984=DIRECTION('ref_axis',(1.,0.,0.));
#15985=DIRECTION('',(0.707106781186546,0.707106781186549,8.65956056235491E-17));
#15986=DIRECTION('center_axis',(0.,-1.,0.));
#15987=DIRECTION('ref_axis',(1.,0.,0.));
#15988=DIRECTION('',(0.707106781186546,0.707106781186549,8.65956056235491E-17));
#15989=DIRECTION('center_axis',(0.,-1.,0.));
#15990=DIRECTION('ref_axis',(1.,0.,0.));
#15991=DIRECTION('',(0.707106781186547,0.707106781186547,8.65956056235493E-17));
#15992=DIRECTION('center_axis',(0.,-1.,0.));
#15993=DIRECTION('ref_axis',(1.,0.,0.));
#15994=DIRECTION('',(0.707106781186547,0.707106781186547,8.65956056235493E-17));
#15995=DIRECTION('center_axis',(0.,-1.,0.));
#15996=DIRECTION('ref_axis',(1.,0.,0.));
#15997=DIRECTION('',(0.707106781186546,0.707106781186549,8.65956056235491E-17));
#15998=DIRECTION('center_axis',(-0.707106781186548,0.,-0.707106781186548));
#15999=DIRECTION('ref_axis',(-0.707106781186548,0.,0.707106781186548));
#16000=DIRECTION('',(0.707106781186548,0.,-0.707106781186548));
#16001=DIRECTION('',(0.,-1.,0.));
#16002=DIRECTION('',(-0.707106781186548,0.,0.707106781186548));
#16003=DIRECTION('center_axis',(1.,0.,0.));
#16004=DIRECTION('ref_axis',(0.,2.96059473233374E-15,-1.));
#16005=DIRECTION('',(0.707106781186548,0.707106781186548,0.));
#16006=DIRECTION('center_axis',(-1.,0.,0.));
#16007=DIRECTION('ref_axis',(0.,2.96059473233374E-15,-1.));
#16008=DIRECTION('center_axis',(-0.707106781186548,0.707106781186548,0.));
#16009=DIRECTION('ref_axis',(0.,0.,1.));
#16010=DIRECTION('',(0.707106781186548,0.707106781186548,-3.14018491736756E-15));
#16011=DIRECTION('',(0.,0.,-1.));
#16012=DIRECTION('center_axis',(1.,0.,0.));
#16013=DIRECTION('ref_axis',(0.,1.,2.22044604925031E-15));
#16014=DIRECTION('',(0.707106781186548,0.,0.707106781186548));
#16015=DIRECTION('center_axis',(-1.,0.,0.));
#16016=DIRECTION('ref_axis',(0.,1.,2.22044604925031E-15));
#16017=DIRECTION('center_axis',(-0.707106781186548,0.,0.707106781186548));
#16018=DIRECTION('ref_axis',(0.707106781186548,0.,0.707106781186548));
#16019=DIRECTION('',(0.707106781186548,-3.14018491736756E-15,0.707106781186548));
#16020=DIRECTION('',(0.,1.,0.));
#16021=DIRECTION('center_axis',(1.,0.,0.));
#16022=DIRECTION('ref_axis',(0.,-1.85037170770859E-15,1.));
#16023=DIRECTION('',(0.707106781186546,-0.707106781186549,3.14018491736755E-15));
#16024=DIRECTION('center_axis',(-1.,0.,0.));
#16025=DIRECTION('ref_axis',(0.,-1.85037170770859E-15,1.));
#16026=DIRECTION('center_axis',(-0.707106781186548,-0.707106781186547,0.));
#16027=DIRECTION('ref_axis',(0.,0.,1.));
#16028=DIRECTION('',(0.707106781186547,-0.707106781186548,3.14018491736756E-15));
#16029=DIRECTION('center_axis',(1.,0.,0.));
#16030=DIRECTION('ref_axis',(0.,-1.,-1.48029736616687E-15));
#16031=DIRECTION('center_axis',(-1.,0.,0.));
#16032=DIRECTION('ref_axis',(0.,-1.,-1.48029736616687E-15));
#16033=DIRECTION('center_axis',(1.,0.,0.));
#16034=DIRECTION('ref_axis',(0.,-1.85037170770859E-15,1.));
#16035=DIRECTION('center_axis',(1.,0.,0.));
#16036=DIRECTION('ref_axis',(0.,-1.85037170770859E-15,1.));
#16037=DIRECTION('',(1.,0.,0.));
#16038=DIRECTION('center_axis',(1.,0.,0.));
#16039=DIRECTION('ref_axis',(0.,-1.,-1.48029736616687E-15));
#16040=DIRECTION('',(1.,0.,0.));
#16041=DIRECTION('center_axis',(1.,0.,0.));
#16042=DIRECTION('ref_axis',(0.,-1.,-1.48029736616687E-15));
#16043=DIRECTION('center_axis',(0.,0.,-1.));
#16044=DIRECTION('ref_axis',(0.,1.,0.));
#16045=DIRECTION('',(1.,0.,0.));
#16046=DIRECTION('',(0.,1.,0.));
#16047=DIRECTION('center_axis',(0.,0.,-1.));
#16048=DIRECTION('ref_axis',(1.,0.,0.));
#16049=DIRECTION('center_axis',(0.,0.,-1.));
#16050=DIRECTION('ref_axis',(1.,0.,0.));
#16051=DIRECTION('center_axis',(0.,0.,-1.));
#16052=DIRECTION('ref_axis',(1.,0.,0.));
#16053=DIRECTION('center_axis',(0.,0.,-1.));
#16054=DIRECTION('ref_axis',(1.,0.,0.));
#16055=DIRECTION('center_axis',(0.,0.,-1.));
#16056=DIRECTION('ref_axis',(1.,0.,0.));
#16057=DIRECTION('center_axis',(0.,0.,-1.));
#16058=DIRECTION('ref_axis',(1.,0.,0.));
#16059=DIRECTION('center_axis',(0.,0.,-1.));
#16060=DIRECTION('ref_axis',(1.,0.,0.));
#16061=DIRECTION('',(0.707106781186547,-8.65956056235493E-17,0.707106781186547));
#16062=DIRECTION('center_axis',(0.,0.,-1.));
#16063=DIRECTION('ref_axis',(1.,0.,0.));
#16064=DIRECTION('',(0.707106781186547,-8.65956056235493E-17,0.707106781186547));
#16065=DIRECTION('center_axis',(0.,0.,-1.));
#16066=DIRECTION('ref_axis',(1.,0.,0.));
#16067=DIRECTION('',(0.707106781186548,-8.65956056235493E-17,0.707106781186548));
#16068=DIRECTION('center_axis',(0.,0.,-1.));
#16069=DIRECTION('ref_axis',(1.,0.,0.));
#16070=DIRECTION('',(0.707106781186549,-8.65956056235495E-17,0.707106781186546));
#16071=DIRECTION('center_axis',(0.,0.,-1.));
#16072=DIRECTION('ref_axis',(1.,0.,0.));
#16073=DIRECTION('',(0.707106781186549,-8.65956056235495E-17,0.707106781186546));
#16074=DIRECTION('center_axis',(0.,0.,-1.));
#16075=DIRECTION('ref_axis',(1.,0.,0.));
#16076=DIRECTION('',(0.707106781186547,-8.65956056235493E-17,0.707106781186547));
#16077=DIRECTION('center_axis',(0.707106781186534,-0.707106781186561,0.));
#16078=DIRECTION('ref_axis',(0.,0.,-1.));
#16079=DIRECTION('',(0.707106781186561,0.707106781186534,-2.61682076447291E-15));
#16080=DIRECTION('',(0.,0.,1.));
#16081=DIRECTION('',(-0.707106781186563,-0.707106781186532,0.));
#16082=DIRECTION('center_axis',(-1.,0.,0.));
#16083=DIRECTION('ref_axis',(0.,-1.,-1.48029736616687E-15));
#16084=DIRECTION('',(0.707106781186561,2.61682076447291E-15,0.707106781186534));
#16085=DIRECTION('center_axis',(-1.,0.,0.));
#16086=DIRECTION('ref_axis',(0.,-1.,-1.48029736616687E-15));
#16087=DIRECTION('center_axis',(0.707106781186534,0.,-0.707106781186561));
#16088=DIRECTION('ref_axis',(-0.707106781186561,0.,-0.707106781186534));
#16089=DIRECTION('',(0.707106781186561,0.,0.707106781186534));
#16090=DIRECTION('',(0.,-1.,0.));
#16091=DIRECTION('center_axis',(-1.,0.,0.));
#16092=DIRECTION('ref_axis',(0.,2.96059473233374E-15,-1.));
#16093=DIRECTION('',(0.707106781186563,-0.707106781186532,0.));
#16094=DIRECTION('center_axis',(-1.,0.,0.));
#16095=DIRECTION('ref_axis',(0.,2.96059473233374E-15,-1.));
#16096=DIRECTION('center_axis',(1.,0.,0.));
#16097=DIRECTION('ref_axis',(0.,2.96059473233374E-15,-1.));
#16098=DIRECTION('center_axis',(0.707106781186532,0.707106781186563,0.));
#16099=DIRECTION('ref_axis',(0.,0.,-1.));
#16100=DIRECTION('',(0.707106781186563,-0.707106781186532,2.61682076447292E-15));
#16101=DIRECTION('',(0.,0.,-1.));
#16102=DIRECTION('',(0.,0.,1.));
#16103=DIRECTION('center_axis',(-1.,0.,0.));
#16104=DIRECTION('ref_axis',(0.,1.,2.22044604925031E-15));
#16105=DIRECTION('',(0.707106781186563,0.,-0.707106781186532));
#16106=DIRECTION('center_axis',(-1.,0.,0.));
#16107=DIRECTION('ref_axis',(0.,1.,2.22044604925031E-15));
#16108=DIRECTION('center_axis',(1.,0.,0.));
#16109=DIRECTION('ref_axis',(0.,1.,2.22044604925031E-15));
#16110=DIRECTION('center_axis',(0.707106781186534,0.,0.707106781186561));
#16111=DIRECTION('ref_axis',(0.707106781186561,0.,-0.707106781186534));
#16112=DIRECTION('',(0.707106781186561,2.61682076447291E-15,-0.707106781186534));
#16113=DIRECTION('',(0.,1.,0.));
#16114=DIRECTION('',(0.,-1.,0.));
#16115=DIRECTION('center_axis',(-1.,0.,0.));
#16116=DIRECTION('ref_axis',(0.,-1.85037170770859E-15,1.));
#16117=DIRECTION('center_axis',(-1.,0.,0.));
#16118=DIRECTION('ref_axis',(0.,-1.85037170770859E-15,1.));
#16119=DIRECTION('center_axis',(1.,0.,0.));
#16120=DIRECTION('ref_axis',(0.,2.96059473233374E-15,-1.));
#16121=DIRECTION('',(1.,0.,0.));
#16122=DIRECTION('center_axis',(1.,0.,0.));
#16123=DIRECTION('ref_axis',(0.,0.,-1.));
#16124=DIRECTION('',(0.,1.,0.));
#16125=DIRECTION('center_axis',(1.,0.,0.));
#16126=DIRECTION('ref_axis',(0.,-1.,0.));
#16127=DIRECTION('',(0.,0.,-1.));
#16128=DIRECTION('center_axis',(1.,0.,0.));
#16129=DIRECTION('ref_axis',(0.,1.79429983777803E-15,1.));
#16130=DIRECTION('',(0.,-1.,0.));
#16131=DIRECTION('center_axis',(1.,0.,0.));
#16132=DIRECTION('ref_axis',(0.,1.,1.79429983777804E-15));
#16133=DIRECTION('',(0.,0.,1.));
#16134=DIRECTION('center_axis',(1.,0.,0.));
#16135=DIRECTION('ref_axis',(0.,-7.17719935111212E-15,-1.));
#16136=DIRECTION('center_axis',(0.707106781186534,0.,0.707106781186561));
#16137=DIRECTION('ref_axis',(0.707106781186561,0.,-0.707106781186534));
#16138=DIRECTION('',(0.707106781186561,2.61682076447291E-15,-0.707106781186534));
#16139=DIRECTION('',(-0.707106781186561,0.,0.707106781186534));
#16140=DIRECTION('center_axis',(1.,0.,0.));
#16141=DIRECTION('ref_axis',(0.,-1.,0.));
#16142=DIRECTION('',(0.707106781186561,-0.707106781186534,0.));
#16143=DIRECTION('center_axis',(0.707106781186534,0.707106781186561,0.));
#16144=DIRECTION('ref_axis',(0.,0.,-1.));
#16145=DIRECTION('',(0.707106781186561,-0.707106781186534,2.61682076447291E-15));
#16146=DIRECTION('center_axis',(1.,0.,0.));
#16147=DIRECTION('ref_axis',(0.,1.79429983777803E-15,1.));
#16148=DIRECTION('',(0.707106781186561,0.,0.707106781186534));
#16149=DIRECTION('center_axis',(-1.,0.,0.));
#16150=DIRECTION('ref_axis',(0.,1.79429983777803E-15,1.));
#16151=DIRECTION('center_axis',(0.707106781186534,0.,-0.707106781186561));
#16152=DIRECTION('ref_axis',(-0.707106781186561,0.,-0.707106781186534));
#16153=DIRECTION('',(0.707106781186555,0.,0.70710678118654));
#16154=DIRECTION('',(0.,1.,0.));
#16155=DIRECTION('center_axis',(1.,0.,0.));
#16156=DIRECTION('ref_axis',(0.,1.,1.79429983777804E-15));
#16157=DIRECTION('',(0.707106781186563,0.707106781186532,0.));
#16158=DIRECTION('center_axis',(-1.,0.,0.));
#16159=DIRECTION('ref_axis',(0.,1.,1.79429983777804E-15));
#16160=DIRECTION('center_axis',(0.707106781186532,-0.707106781186563,0.));
#16161=DIRECTION('ref_axis',(0.,0.,-1.));
#16162=DIRECTION('',(0.707106781186568,0.707106781186527,-2.61682076447294E-15));
#16163=DIRECTION('',(0.,0.,-1.));
#16164=DIRECTION('center_axis',(1.,0.,0.));
#16165=DIRECTION('ref_axis',(0.,-7.17719935111212E-15,-1.));
#16166=DIRECTION('center_axis',(1.,0.,0.));
#16167=DIRECTION('ref_axis',(0.,1.79429983777803E-15,1.));
#16168=DIRECTION('',(1.,0.,0.));
#16169=DIRECTION('center_axis',(0.,-1.,0.));
#16170=DIRECTION('ref_axis',(0.,0.,-1.));
#16171=DIRECTION('',(1.,0.,0.));
#16172=DIRECTION('center_axis',(1.,0.,0.));
#16173=DIRECTION('ref_axis',(0.,1.,1.79429983777804E-15));
#16174=DIRECTION('',(1.,0.,0.));
#16175=DIRECTION('center_axis',(0.,0.,-1.));
#16176=DIRECTION('ref_axis',(0.,1.,0.));
#16177=DIRECTION('center_axis',(0.,0.,1.));
#16178=DIRECTION('ref_axis',(0.,-1.,0.));
#16179=DIRECTION('',(1.,0.,0.));
#16180=DIRECTION('center_axis',(1.,0.,0.));
#16181=DIRECTION('ref_axis',(0.,1.,2.22044604925031E-15));
#16182=DIRECTION('',(1.,0.,0.));
#16183=DIRECTION('center_axis',(0.,1.,0.));
#16184=DIRECTION('ref_axis',(0.,0.,1.));
#22232=CARTESIAN_POINT('',(0.,0.,0.));
#22233=CARTESIAN_POINT('Origin',(46.95,31.75,-20.8875));
#22234=CARTESIAN_POINT('',(41.25,31.75,-20.6375));
#22235=CARTESIAN_POINT('Origin',(46.95,31.75,-20.6375));
#22236=CARTESIAN_POINT('',(41.75,31.75,-21.1375));
#22237=CARTESIAN_POINT('',(41.5,31.75,-20.8875));
#22238=CARTESIAN_POINT('Origin',(46.95,31.75,-21.1375));
#22239=CARTESIAN_POINT('Origin',(-67.35,51.15,-20.6375));
#22240=CARTESIAN_POINT('',(-66.85,12.35,-20.6375));
#22241=CARTESIAN_POINT('',(-66.85,51.15,-20.6375));
#22242=CARTESIAN_POINT('',(-66.85,41.45,-20.6375));
#22243=CARTESIAN_POINT('',(109.85,12.35,-20.6375));
#22244=CARTESIAN_POINT('',(-67.35,12.35,-20.6375));
#22245=CARTESIAN_POINT('',(109.85,51.15,-20.6375));
#22246=CARTESIAN_POINT('',(109.85,41.45,-20.6375));
#22247=CARTESIAN_POINT('',(-67.35,51.15,-20.6375));
#22248=CARTESIAN_POINT('',(-22.25,31.75,-20.6375));
#22249=CARTESIAN_POINT('Origin',(-16.55,31.75,-20.6375));
#22250=CARTESIAN_POINT('',(9.50000000000001,31.75,-20.6375));
#22251=CARTESIAN_POINT('Origin',(15.2,31.75,-20.6375));
#22252=CARTESIAN_POINT('',(57.125,31.75,-20.6375));
#22253=CARTESIAN_POINT('Origin',(62.825,31.75,-20.6375));
#22254=CARTESIAN_POINT('',(25.375,31.75,-20.6375));
#22255=CARTESIAN_POINT('Origin',(31.075,31.75,-20.6375));
#22256=CARTESIAN_POINT('',(-6.375,31.75,-20.6375));
#22257=CARTESIAN_POINT('Origin',(-0.674999999999997,31.75,-20.6375));
#22258=CARTESIAN_POINT('Origin',(46.95,31.75,-25.4));
#22259=CARTESIAN_POINT('',(41.75,31.75,-24.9));
#22260=CARTESIAN_POINT('Origin',(46.95,31.75,-24.9));
#22261=CARTESIAN_POINT('',(41.75,31.75,-25.4));
#22262=CARTESIAN_POINT('Origin',(-16.55,31.75,-20.8875));
#22263=CARTESIAN_POINT('',(-21.75,31.75,-21.1375));
#22264=CARTESIAN_POINT('',(-22.,31.75,-20.8875));
#22265=CARTESIAN_POINT('Origin',(-16.55,31.75,-21.1375));
#22266=CARTESIAN_POINT('Origin',(-16.55,31.75,-25.4));
#22267=CARTESIAN_POINT('',(-21.75,31.75,-24.9));
#22268=CARTESIAN_POINT('Origin',(-16.55,31.75,-24.9));
#22269=CARTESIAN_POINT('',(-21.75,31.75,-25.4));
#22270=CARTESIAN_POINT('Origin',(-0.674999999999997,31.75,-20.8875));
#22271=CARTESIAN_POINT('',(-5.875,31.75,-21.1375));
#22272=CARTESIAN_POINT('',(-6.125,31.75,-20.8875));
#22273=CARTESIAN_POINT('Origin',(-0.674999999999997,31.75,-21.1375));
#22274=CARTESIAN_POINT('Origin',(-0.674999999999997,31.75,-25.4));
#22275=CARTESIAN_POINT('',(-5.875,31.75,-24.9));
#22276=CARTESIAN_POINT('Origin',(-0.674999999999997,31.75,-24.9));
#22277=CARTESIAN_POINT('',(-5.875,31.75,-25.4));
#22278=CARTESIAN_POINT('Origin',(15.2,31.75,-20.8875));
#22279=CARTESIAN_POINT('',(10.,31.75,-21.1375));
#22280=CARTESIAN_POINT('',(9.75000000000001,31.75,-20.8875));
#22281=CARTESIAN_POINT('Origin',(15.2,31.75,-21.1375));
#22282=CARTESIAN_POINT('Origin',(15.2,31.75,-25.4));
#22283=CARTESIAN_POINT('',(10.,31.75,-24.9));
#22284=CARTESIAN_POINT('Origin',(15.2,31.75,-24.9));
#22285=CARTESIAN_POINT('',(10.,31.75,-25.4));
#22286=CARTESIAN_POINT('Origin',(31.075,31.75,-20.8875));
#22287=CARTESIAN_POINT('',(25.875,31.75,-21.1375));
#22288=CARTESIAN_POINT('',(25.625,31.75,-20.8875));
#22289=CARTESIAN_POINT('Origin',(31.075,31.75,-21.1375));
#22290=CARTESIAN_POINT('Origin',(31.075,31.75,-25.4));
#22291=CARTESIAN_POINT('',(25.875,31.75,-24.9));
#22292=CARTESIAN_POINT('Origin',(31.075,31.75,-24.9));
#22293=CARTESIAN_POINT('',(25.875,31.75,-25.4));
#22294=CARTESIAN_POINT('Origin',(62.825,31.75,-20.8875));
#22295=CARTESIAN_POINT('',(57.625,31.75,-21.1375));
#22296=CARTESIAN_POINT('',(57.375,31.75,-20.8875));
#22297=CARTESIAN_POINT('Origin',(62.825,31.75,-21.1375));
#22298=CARTESIAN_POINT('Origin',(62.825,31.75,-25.4));
#22299=CARTESIAN_POINT('',(57.625,31.75,-24.9));
#22300=CARTESIAN_POINT('Origin',(62.825,31.75,-24.9));
#22301=CARTESIAN_POINT('',(57.625,31.75,-25.4));
#22302=CARTESIAN_POINT('Origin',(62.825,10.8625,0.));
#22303=CARTESIAN_POINT('',(57.125,11.1125,6.98048675513991E-16));
#22304=CARTESIAN_POINT('Origin',(62.825,11.1125,0.));
#22305=CARTESIAN_POINT('',(57.625,10.6125,-6.36816335556623E-16));
#22306=CARTESIAN_POINT('',(57.375,10.8625,6.67432505535307E-16));
#22307=CARTESIAN_POINT('Origin',(62.825,10.6125,0.));
#22308=CARTESIAN_POINT('Origin',(-67.35,11.1125,-19.4));
#22309=CARTESIAN_POINT('',(-66.85,11.1125,19.4));
#22310=CARTESIAN_POINT('',(-66.85,11.1125,-19.4));
#22311=CARTESIAN_POINT('',(-66.85,11.1125,-9.7));
#22312=CARTESIAN_POINT('',(109.85,11.1125,19.4));
#22313=CARTESIAN_POINT('',(-67.35,11.1125,19.4));
#22314=CARTESIAN_POINT('',(109.85,11.1125,-19.4));
#22315=CARTESIAN_POINT('',(109.85,11.1125,-9.7));
#22316=CARTESIAN_POINT('',(-67.35,11.1125,-19.4));
#22317=CARTESIAN_POINT('',(25.375,11.1125,6.98048675513991E-16));
#22318=CARTESIAN_POINT('Origin',(31.075,11.1125,0.));
#22319=CARTESIAN_POINT('',(-6.375,11.1125,6.98048675513991E-16));
#22320=CARTESIAN_POINT('Origin',(-0.674999999999997,11.1125,0.));
#22321=CARTESIAN_POINT('',(41.25,11.1125,6.98048675513991E-16));
#22322=CARTESIAN_POINT('Origin',(46.95,11.1125,0.));
#22323=CARTESIAN_POINT('',(-22.25,11.1125,6.98048675513991E-16));
#22324=CARTESIAN_POINT('Origin',(-16.55,11.1125,0.));
#22325=CARTESIAN_POINT('',(9.50000000000001,11.1125,6.98048675513991E-16));
#22326=CARTESIAN_POINT('Origin',(15.2,11.1125,0.));
#22327=CARTESIAN_POINT('',(-56.8,11.1125,1.04094977927525E-15));
#22328=CARTESIAN_POINT('Origin',(-48.3,11.1125,0.));
#22329=CARTESIAN_POINT('Origin',(62.825,6.35,0.));
#22330=CARTESIAN_POINT('',(57.625,6.85,6.36816335556623E-16));
#22331=CARTESIAN_POINT('Origin',(62.825,6.85,0.));
#22332=CARTESIAN_POINT('',(57.625,6.35,6.36816335556623E-16));
#22333=CARTESIAN_POINT('Origin',(-67.1,10.8625,-9.7));
#22334=CARTESIAN_POINT('',(-67.35,10.6125,19.4));
#22335=CARTESIAN_POINT('',(-67.35,10.6125,19.4));
#22336=CARTESIAN_POINT('',(-67.35,10.6125,-19.4));
#22337=CARTESIAN_POINT('',(-66.85,11.1125,-19.4));
#22338=CARTESIAN_POINT('',(-67.35,10.6125,-9.7));
#22339=CARTESIAN_POINT('Origin',(-67.1,12.35,19.4));
#22340=CARTESIAN_POINT('',(-67.35,12.35,21.1375));
#22341=CARTESIAN_POINT('',(-66.85,12.35,20.6375));
#22342=CARTESIAN_POINT('',(-67.35,12.35,21.1375));
#22343=CARTESIAN_POINT('Origin',(-66.85,12.35,19.4));
#22344=CARTESIAN_POINT('Origin',(-67.35,12.35,19.4));
#22345=CARTESIAN_POINT('Origin',(-67.1,22.05,20.8875));
#22346=CARTESIAN_POINT('',(-67.35,51.15,21.1375));
#22347=CARTESIAN_POINT('',(-66.85,51.15,20.6375));
#22348=CARTESIAN_POINT('',(-67.35,51.15,21.1375));
#22349=CARTESIAN_POINT('',(-66.85,22.05,20.6375));
#22350=CARTESIAN_POINT('',(-67.35,22.05,21.1375));
#22351=CARTESIAN_POINT('Origin',(-67.1,51.15,19.4));
#22352=CARTESIAN_POINT('',(-67.35,52.8875,19.4));
#22353=CARTESIAN_POINT('',(-66.85,52.3875,19.4));
#22354=CARTESIAN_POINT('',(-67.35,52.8875,19.4));
#22355=CARTESIAN_POINT('Origin',(-66.85,51.15,19.4));
#22356=CARTESIAN_POINT('Origin',(-67.35,51.15,19.4));
#22357=CARTESIAN_POINT('Origin',(-67.1,52.6375,9.7));
#22358=CARTESIAN_POINT('',(-67.35,52.8875,-19.4));
#22359=CARTESIAN_POINT('',(-66.85,52.3875,-19.4));
#22360=CARTESIAN_POINT('',(-67.35,52.8875,-19.4));
#22361=CARTESIAN_POINT('',(-66.85,52.3875,9.7));
#22362=CARTESIAN_POINT('',(-67.35,52.8875,9.7));
#22363=CARTESIAN_POINT('Origin',(-67.1,51.15,-19.4));
#22364=CARTESIAN_POINT('',(-67.35,51.15,-21.1375));
#22365=CARTESIAN_POINT('',(-67.35,51.15,-21.1375));
#22366=CARTESIAN_POINT('Origin',(-66.85,51.15,-19.4));
#22367=CARTESIAN_POINT('Origin',(-67.35,51.15,-19.4));
#22368=CARTESIAN_POINT('Origin',(-67.1,41.45,-20.8875));
#22369=CARTESIAN_POINT('',(-67.35,12.35,-21.1375));
#22370=CARTESIAN_POINT('',(-67.35,12.35,-21.1375));
#22371=CARTESIAN_POINT('',(-67.35,41.45,-21.1375));
#22372=CARTESIAN_POINT('Origin',(-67.1,12.35,-19.4));
#22373=CARTESIAN_POINT('Origin',(-66.85,12.35,-19.4));
#22374=CARTESIAN_POINT('Origin',(-67.35,12.35,-19.4));
#22375=CARTESIAN_POINT('Origin',(-67.35,51.15,-19.4));
#22376=CARTESIAN_POINT('',(109.85,52.3875,-19.4));
#22377=CARTESIAN_POINT('Origin',(109.85,51.15,-19.4));
#22378=CARTESIAN_POINT('',(-67.35,52.3875,-19.4));
#22379=CARTESIAN_POINT('Origin',(-67.35,12.35,-19.4));
#22380=CARTESIAN_POINT('Origin',(109.85,12.35,-19.4));
#22381=CARTESIAN_POINT('Origin',(-67.35,31.75,0.));
#22382=CARTESIAN_POINT('',(-67.35,12.35,-24.9));
#22383=CARTESIAN_POINT('',(-67.35,51.15,-24.9));
#22384=CARTESIAN_POINT('',(-67.35,22.05,-24.9));
#22385=CARTESIAN_POINT('',(-67.35,6.85,-19.4));
#22386=CARTESIAN_POINT('Origin',(-67.35,12.35,-19.4));
#22387=CARTESIAN_POINT('',(-67.35,6.85,19.4));
#22388=CARTESIAN_POINT('',(-67.35,6.85,9.7));
#22389=CARTESIAN_POINT('',(-67.35,12.35,24.9));
#22390=CARTESIAN_POINT('Origin',(-67.35,12.35,19.4));
#22391=CARTESIAN_POINT('',(-67.35,51.15,24.9));
#22392=CARTESIAN_POINT('',(-67.35,41.45,24.9));
#22393=CARTESIAN_POINT('',(-67.35,56.65,19.4));
#22394=CARTESIAN_POINT('Origin',(-67.35,51.15,19.4));
#22395=CARTESIAN_POINT('',(-67.35,56.65,-19.4));
#22396=CARTESIAN_POINT('',(-67.35,56.65,-9.7));
#22397=CARTESIAN_POINT('Origin',(-67.35,51.15,-19.4));
#22398=CARTESIAN_POINT('Origin',(-48.3,10.8625,0.));
#22399=CARTESIAN_POINT('',(-56.3,10.6125,-9.79717439317882E-16));
#22400=CARTESIAN_POINT('',(-56.55,10.8625,1.01033360929657E-15));
#22401=CARTESIAN_POINT('Origin',(-48.3,10.6125,0.));
#22402=CARTESIAN_POINT('Origin',(-48.3,6.35,0.));
#22403=CARTESIAN_POINT('',(-56.3,6.85,9.79717439317882E-16));
#22404=CARTESIAN_POINT('Origin',(-48.3,6.85,0.));
#22405=CARTESIAN_POINT('',(-56.3,6.35,9.79717439317882E-16));
#22406=CARTESIAN_POINT('Origin',(31.075,10.8625,0.));
#22407=CARTESIAN_POINT('',(25.875,10.6125,-6.36816335556624E-16));
#22408=CARTESIAN_POINT('',(25.625,10.8625,6.67432505535307E-16));
#22409=CARTESIAN_POINT('Origin',(31.075,10.6125,0.));
#22410=CARTESIAN_POINT('Origin',(31.075,6.35,0.));
#22411=CARTESIAN_POINT('',(25.875,6.85,6.36816335556624E-16));
#22412=CARTESIAN_POINT('Origin',(31.075,6.85,0.));
#22413=CARTESIAN_POINT('',(25.875,6.35,6.36816335556624E-16));
#22414=CARTESIAN_POINT('Origin',(15.2,10.8625,0.));
#22415=CARTESIAN_POINT('',(10.,10.6125,-6.36816335556623E-16));
#22416=CARTESIAN_POINT('',(9.75000000000001,10.8625,6.67432505535307E-16));
#22417=CARTESIAN_POINT('Origin',(15.2,10.6125,0.));
#22418=CARTESIAN_POINT('Origin',(15.2,6.35,0.));
#22419=CARTESIAN_POINT('',(10.,6.85,6.36816335556623E-16));
#22420=CARTESIAN_POINT('Origin',(15.2,6.85,0.));
#22421=CARTESIAN_POINT('',(10.,6.35,6.36816335556623E-16));
#22422=CARTESIAN_POINT('Origin',(-0.674999999999997,10.8625,0.));
#22423=CARTESIAN_POINT('',(-5.875,10.6125,-6.36816335556624E-16));
#22424=CARTESIAN_POINT('',(-6.125,10.8625,6.67432505535308E-16));
#22425=CARTESIAN_POINT('Origin',(-0.674999999999997,10.6125,0.));
#22426=CARTESIAN_POINT('Origin',(-0.674999999999997,6.35,0.));
#22427=CARTESIAN_POINT('',(-5.875,6.85,6.36816335556624E-16));
#22428=CARTESIAN_POINT('Origin',(-0.674999999999997,6.85,0.));
#22429=CARTESIAN_POINT('',(-5.875,6.35,6.36816335556624E-16));
#22430=CARTESIAN_POINT('Origin',(-16.55,10.8625,0.));
#22431=CARTESIAN_POINT('',(-21.75,10.6125,-6.36816335556624E-16));
#22432=CARTESIAN_POINT('',(-22.,10.8625,6.67432505535308E-16));
#22433=CARTESIAN_POINT('Origin',(-16.55,10.6125,0.));
#22434=CARTESIAN_POINT('Origin',(-16.55,6.35,0.));
#22435=CARTESIAN_POINT('',(-21.75,6.85,6.36816335556624E-16));
#22436=CARTESIAN_POINT('Origin',(-16.55,6.85,0.));
#22437=CARTESIAN_POINT('',(-21.75,6.35,6.36816335556624E-16));
#22438=CARTESIAN_POINT('Origin',(46.95,10.8625,0.));
#22439=CARTESIAN_POINT('',(41.75,10.6125,-6.36816335556623E-16));
#22440=CARTESIAN_POINT('',(41.5,10.8625,6.67432505535307E-16));
#22441=CARTESIAN_POINT('Origin',(46.95,10.6125,0.));
#22442=CARTESIAN_POINT('Origin',(46.95,6.35,0.));
#22443=CARTESIAN_POINT('',(41.75,6.85,6.36816335556623E-16));
#22444=CARTESIAN_POINT('Origin',(46.95,6.85,0.));
#22445=CARTESIAN_POINT('',(41.75,6.35,6.36816335556623E-16));
#22446=CARTESIAN_POINT('Origin',(-48.3,6.6,0.));
#22447=CARTESIAN_POINT('',(-56.8,6.35,-1.04094977927525E-15));
#22448=CARTESIAN_POINT('Origin',(-48.3,6.35,0.));
#22449=CARTESIAN_POINT('',(-56.55,6.6,-1.01033360929657E-15));
#22450=CARTESIAN_POINT('Origin',(-67.35,6.35,19.4));
#22451=CARTESIAN_POINT('',(-66.85,6.35,-19.4));
#22452=CARTESIAN_POINT('',(-66.85,6.35,19.4));
#22453=CARTESIAN_POINT('',(-66.85,6.35,9.7));
#22454=CARTESIAN_POINT('',(109.85,6.35,-19.4));
#22455=CARTESIAN_POINT('',(-67.35,6.35,-19.4));
#22456=CARTESIAN_POINT('',(109.85,6.35,19.4));
#22457=CARTESIAN_POINT('',(109.85,6.35,9.7));
#22458=CARTESIAN_POINT('',(-67.35,6.35,19.4));
#22459=CARTESIAN_POINT('',(57.125,6.35,-6.98048675513991E-16));
#22460=CARTESIAN_POINT('Origin',(62.825,6.35,0.));
#22461=CARTESIAN_POINT('',(9.50000000000001,6.35,-6.98048675513991E-16));
#22462=CARTESIAN_POINT('Origin',(15.2,6.35,0.));
#22463=CARTESIAN_POINT('',(-22.25,6.35,-6.98048675513991E-16));
#22464=CARTESIAN_POINT('Origin',(-16.55,6.35,0.));
#22465=CARTESIAN_POINT('',(41.25,6.35,-6.98048675513991E-16));
#22466=CARTESIAN_POINT('Origin',(46.95,6.35,0.));
#22467=CARTESIAN_POINT('',(-6.375,6.35,-6.98048675513991E-16));
#22468=CARTESIAN_POINT('Origin',(-0.674999999999997,6.35,0.));
#22469=CARTESIAN_POINT('',(25.375,6.35,-6.98048675513991E-16));
#22470=CARTESIAN_POINT('Origin',(31.075,6.35,0.));
#22471=CARTESIAN_POINT('Origin',(62.825,6.6,0.));
#22472=CARTESIAN_POINT('',(57.375,6.6,-6.67432505535307E-16));
#22473=CARTESIAN_POINT('Origin',(31.075,6.6,0.));
#22474=CARTESIAN_POINT('',(25.625,6.6,-6.67432505535307E-16));
#22475=CARTESIAN_POINT('Origin',(15.2,6.6,0.));
#22476=CARTESIAN_POINT('',(9.75000000000001,6.6,-6.67432505535307E-16));
#22477=CARTESIAN_POINT('Origin',(-0.674999999999997,6.6,0.));
#22478=CARTESIAN_POINT('',(-6.125,6.6,-6.67432505535308E-16));
#22479=CARTESIAN_POINT('Origin',(-16.55,6.6,0.));
#22480=CARTESIAN_POINT('',(-22.,6.6,-6.67432505535308E-16));
#22481=CARTESIAN_POINT('Origin',(46.95,6.6,0.));
#22482=CARTESIAN_POINT('',(41.5,6.6,-6.67432505535307E-16));
#22483=CARTESIAN_POINT('Origin',(-67.1,22.05,-25.15));
#22484=CARTESIAN_POINT('',(-66.85,51.15,-25.4));
#22485=CARTESIAN_POINT('',(-67.35,51.15,-24.9));
#22486=CARTESIAN_POINT('',(-66.85,12.35,-25.4));
#22487=CARTESIAN_POINT('',(-66.85,22.05,-25.4));
#22488=CARTESIAN_POINT('',(-66.85,12.35,-25.4));
#22489=CARTESIAN_POINT('Origin',(-67.1,51.15,-19.4));
#22490=CARTESIAN_POINT('',(-66.85,57.15,-19.4));
#22491=CARTESIAN_POINT('',(-67.35,56.65,-19.4));
#22492=CARTESIAN_POINT('Origin',(-66.85,51.15,-19.4));
#22493=CARTESIAN_POINT('Origin',(-67.1,56.9,-9.7));
#22494=CARTESIAN_POINT('',(-66.85,57.15,19.4));
#22495=CARTESIAN_POINT('',(-67.35,56.65,19.4));
#22496=CARTESIAN_POINT('',(-66.85,57.15,-9.7));
#22497=CARTESIAN_POINT('Origin',(-67.1,51.15,19.4));
#22498=CARTESIAN_POINT('',(-66.85,51.15,25.4));
#22499=CARTESIAN_POINT('',(-67.35,51.15,24.9));
#22500=CARTESIAN_POINT('Origin',(-66.85,51.15,19.4));
#22501=CARTESIAN_POINT('Origin',(-67.1,41.45,25.15));
#22502=CARTESIAN_POINT('',(-66.85,12.35,25.4));
#22503=CARTESIAN_POINT('',(-67.35,12.35,24.9));
#22504=CARTESIAN_POINT('',(-66.85,41.45,25.4));
#22505=CARTESIAN_POINT('Origin',(-67.1,12.35,19.4));
#22506=CARTESIAN_POINT('',(-67.35,6.85,19.4));
#22507=CARTESIAN_POINT('Origin',(-66.85,12.35,19.4));
#22508=CARTESIAN_POINT('Origin',(-67.1,6.6,9.7));
#22509=CARTESIAN_POINT('',(-67.35,6.85,-19.4));
#22510=CARTESIAN_POINT('Origin',(-67.1,12.35,-19.4));
#22511=CARTESIAN_POINT('Origin',(-66.85,12.35,-19.4));
#22512=CARTESIAN_POINT('Origin',(-67.35,12.35,19.4));
#22513=CARTESIAN_POINT('',(109.85,12.35,25.4));
#22514=CARTESIAN_POINT('Origin',(109.85,12.35,19.4));
#22515=CARTESIAN_POINT('',(-67.35,12.35,25.4));
#22516=CARTESIAN_POINT('Origin',(-67.35,12.35,-19.4));
#22517=CARTESIAN_POINT('',(109.85,12.35,-25.4));
#22518=CARTESIAN_POINT('',(-67.35,12.35,-25.4));
#22519=CARTESIAN_POINT('Origin',(109.85,12.35,-19.4));
#22520=CARTESIAN_POINT('Origin',(-67.35,12.35,-25.4));
#22521=CARTESIAN_POINT('',(109.85,51.15,-25.4));
#22522=CARTESIAN_POINT('',(-67.35,51.15,-25.4));
#22523=CARTESIAN_POINT('',(109.85,22.05,-25.4));
#22524=CARTESIAN_POINT('',(57.125,31.75,-25.4));
#22525=CARTESIAN_POINT('Origin',(62.825,31.75,-25.4));
#22526=CARTESIAN_POINT('',(9.50000000000001,31.75,-25.4));
#22527=CARTESIAN_POINT('Origin',(15.2,31.75,-25.4));
#22528=CARTESIAN_POINT('',(-22.25,31.75,-25.4));
#22529=CARTESIAN_POINT('Origin',(-16.55,31.75,-25.4));
#22530=CARTESIAN_POINT('',(41.25,31.75,-25.4));
#22531=CARTESIAN_POINT('Origin',(46.95,31.75,-25.4));
#22532=CARTESIAN_POINT('',(-6.375,31.75,-25.4));
#22533=CARTESIAN_POINT('Origin',(-0.674999999999997,31.75,-25.4));
#22534=CARTESIAN_POINT('',(25.375,31.75,-25.4));
#22535=CARTESIAN_POINT('Origin',(31.075,31.75,-25.4));
#22536=CARTESIAN_POINT('Origin',(62.825,31.75,-25.15));
#22537=CARTESIAN_POINT('',(57.375,31.75,-25.15));
#22538=CARTESIAN_POINT('Origin',(31.075,31.75,-25.15));
#22539=CARTESIAN_POINT('',(25.625,31.75,-25.15));
#22540=CARTESIAN_POINT('Origin',(15.2,31.75,-25.15));
#22541=CARTESIAN_POINT('',(9.75000000000001,31.75,-25.15));
#22542=CARTESIAN_POINT('Origin',(-0.674999999999997,31.75,-25.15));
#22543=CARTESIAN_POINT('',(-6.125,31.75,-25.15));
#22544=CARTESIAN_POINT('Origin',(-16.55,31.75,-25.15));
#22545=CARTESIAN_POINT('',(-22.,31.75,-25.15));
#22546=CARTESIAN_POINT('Origin',(46.95,31.75,-25.15));
#22547=CARTESIAN_POINT('',(41.5,31.75,-25.15));
#22548=CARTESIAN_POINT('Origin',(110.15,6.65,9.7));
#22549=CARTESIAN_POINT('',(110.45,6.95,-19.4));
#22550=CARTESIAN_POINT('',(109.85,6.35,-19.4));
#22551=CARTESIAN_POINT('',(110.45,6.95,19.4));
#22552=CARTESIAN_POINT('',(110.45,6.95,9.7));
#22553=CARTESIAN_POINT('',(110.45,6.95,19.4));
#22554=CARTESIAN_POINT('Origin',(110.15,12.35,-19.4));
#22555=CARTESIAN_POINT('',(110.45,12.35,-24.8));
#22556=CARTESIAN_POINT('',(109.85,12.35,-25.4));
#22557=CARTESIAN_POINT('Origin',(110.45,12.35,-19.4));
#22558=CARTESIAN_POINT('Origin',(110.15,22.05,-25.1));
#22559=CARTESIAN_POINT('',(110.45,51.15,-24.8));
#22560=CARTESIAN_POINT('',(109.85,51.15,-25.4));
#22561=CARTESIAN_POINT('',(110.45,22.05,-24.8));
#22562=CARTESIAN_POINT('Origin',(110.15,51.15,-19.4));
#22563=CARTESIAN_POINT('',(109.85,57.15,-19.4));
#22564=CARTESIAN_POINT('',(110.45,56.55,-19.4));
#22565=CARTESIAN_POINT('',(109.85,57.15,-19.4));
#22566=CARTESIAN_POINT('Origin',(110.45,51.15,-19.4));
#22567=CARTESIAN_POINT('Origin',(109.85,51.15,-19.4));
#22568=CARTESIAN_POINT('Origin',(110.15,56.85,-9.7));
#22569=CARTESIAN_POINT('',(109.85,57.15,19.4));
#22570=CARTESIAN_POINT('',(110.45,56.55,19.4));
#22571=CARTESIAN_POINT('',(109.85,57.15,19.4));
#22572=CARTESIAN_POINT('',(110.45,56.55,-9.7));
#22573=CARTESIAN_POINT('',(109.85,57.15,-9.7));
#22574=CARTESIAN_POINT('Origin',(110.15,51.15,19.4));
#22575=CARTESIAN_POINT('',(109.85,51.15,25.4));
#22576=CARTESIAN_POINT('',(110.45,51.15,24.8));
#22577=CARTESIAN_POINT('',(109.85,51.15,25.4));
#22578=CARTESIAN_POINT('Origin',(110.45,51.15,19.4));
#22579=CARTESIAN_POINT('Origin',(109.85,51.15,19.4));
#22580=CARTESIAN_POINT('Origin',(110.15,41.45,25.1));
#22581=CARTESIAN_POINT('',(110.45,12.35,24.8));
#22582=CARTESIAN_POINT('',(109.85,12.35,25.4));
#22583=CARTESIAN_POINT('',(110.45,41.45,24.8));
#22584=CARTESIAN_POINT('',(109.85,41.45,25.4));
#22585=CARTESIAN_POINT('Origin',(110.15,12.35,19.4));
#22586=CARTESIAN_POINT('Origin',(110.45,12.35,19.4));
#22587=CARTESIAN_POINT('Origin',(-67.35,51.15,-19.4));
#22588=CARTESIAN_POINT('',(-67.35,57.15,-19.4));
#22589=CARTESIAN_POINT('Origin',(110.45,31.75,0.));
#22590=CARTESIAN_POINT('',(110.45,12.35,-21.2375));
#22591=CARTESIAN_POINT('',(110.45,51.15,-21.2375));
#22592=CARTESIAN_POINT('',(110.45,41.45,-21.2375));
#22593=CARTESIAN_POINT('',(110.45,10.5125,-19.4));
#22594=CARTESIAN_POINT('Origin',(110.45,12.35,-19.4));
#22595=CARTESIAN_POINT('',(110.45,10.5125,19.4));
#22596=CARTESIAN_POINT('',(110.45,10.5125,-9.7));
#22597=CARTESIAN_POINT('',(110.45,12.35,21.2375));
#22598=CARTESIAN_POINT('Origin',(110.45,12.35,19.4));
#22599=CARTESIAN_POINT('',(110.45,51.15,21.2375));
#22600=CARTESIAN_POINT('',(110.45,22.05,21.2375));
#22601=CARTESIAN_POINT('',(110.45,52.9875,19.4));
#22602=CARTESIAN_POINT('Origin',(110.45,51.15,19.4));
#22603=CARTESIAN_POINT('',(110.45,52.9875,-19.4));
#22604=CARTESIAN_POINT('',(110.45,52.9875,9.7));
#22605=CARTESIAN_POINT('Origin',(110.45,51.15,-19.4));
#22606=CARTESIAN_POINT('Origin',(110.15,41.45,-20.9375));
#22607=CARTESIAN_POINT('',(109.85,12.35,-20.6375));
#22608=CARTESIAN_POINT('',(110.45,51.15,-21.2375));
#22609=CARTESIAN_POINT('Origin',(110.15,12.35,-19.4));
#22610=CARTESIAN_POINT('',(109.85,11.1125,-19.4));
#22611=CARTESIAN_POINT('Origin',(110.15,10.8125,-9.7));
#22612=CARTESIAN_POINT('',(109.85,11.1125,19.4));
#22613=CARTESIAN_POINT('Origin',(110.15,12.35,19.4));
#22614=CARTESIAN_POINT('',(109.85,12.35,20.6375));
#22615=CARTESIAN_POINT('',(109.85,12.35,20.6375));
#22616=CARTESIAN_POINT('Origin',(109.85,12.35,19.4));
#22617=CARTESIAN_POINT('Origin',(110.15,22.05,20.9375));
#22618=CARTESIAN_POINT('',(109.85,51.15,20.6375));
#22619=CARTESIAN_POINT('',(109.85,51.15,20.6375));
#22620=CARTESIAN_POINT('',(109.85,22.05,20.6375));
#22621=CARTESIAN_POINT('Origin',(110.15,51.15,19.4));
#22622=CARTESIAN_POINT('',(109.85,52.3875,19.4));
#22623=CARTESIAN_POINT('',(109.85,52.3875,19.4));
#22624=CARTESIAN_POINT('Origin',(109.85,51.15,19.4));
#22625=CARTESIAN_POINT('Origin',(110.15,52.6875,9.7));
#22626=CARTESIAN_POINT('',(109.85,52.3875,-19.4));
#22627=CARTESIAN_POINT('',(109.85,52.3875,9.7));
#22628=CARTESIAN_POINT('Origin',(110.15,51.15,-19.4));
#22629=CARTESIAN_POINT('Origin',(-67.35,12.35,19.4));
#22630=CARTESIAN_POINT('',(-67.35,12.35,20.6375));
#22631=CARTESIAN_POINT('Origin',(-67.35,52.3875,19.4));
#22632=CARTESIAN_POINT('',(-67.35,52.3875,19.4));
#22633=CARTESIAN_POINT('Origin',(-67.35,51.15,19.4));
#22634=CARTESIAN_POINT('',(-67.35,51.15,20.6375));
#22635=CARTESIAN_POINT('Origin',(-67.35,12.35,20.6375));
#22636=CARTESIAN_POINT('Origin',(-67.35,51.15,25.4));
#22637=CARTESIAN_POINT('',(-67.35,51.15,25.4));
#22638=CARTESIAN_POINT('Origin',(-67.35,51.15,19.4));
#22639=CARTESIAN_POINT('',(-67.35,57.15,19.4));
#22640=CARTESIAN_POINT('Origin',(-67.35,57.15,-19.4));
#32283=UNCERTAINTY_MEASURE_WITH_UNIT(LENGTH_MEASURE(0.01),#32310,
'DISTANCE_ACCURACY_VALUE',
'Maximum model space distance between geometric entities at asserted c
onnectivities');
#32293=UNCERTAINTY_MEASURE_WITH_UNIT(LENGTH_MEASURE(0.01),#32310,
'DISTANCE_ACCURACY_VALUE',
'Maximum model space distance between geometric entities at asserted c
onnectivities');
#32299=(
GEOMETRIC_REPRESENTATION_CONTEXT(3)
GLOBAL_UNCERTAINTY_ASSIGNED_CONTEXT((#32283))
GLOBAL_UNIT_ASSIGNED_CONTEXT((#32310,#32312,#32313))
REPRESENTATION_CONTEXT('','3D')
);
#32309=(
GEOMETRIC_REPRESENTATION_CONTEXT(3)
GLOBAL_UNCERTAINTY_ASSIGNED_CONTEXT((#32293))
GLOBAL_UNIT_ASSIGNED_CONTEXT((#32310,#32312,#32313))
REPRESENTATION_CONTEXT('','3D')
);
#32310=(
LENGTH_UNIT()
NAMED_UNIT(*)
SI_UNIT(.MILLI.,.METRE.)
);
#32312=(
NAMED_UNIT(*)
PLANE_ANGLE_UNIT()
SI_UNIT($,.RADIAN.)
);
#32313=(
NAMED_UNIT(*)
SI_UNIT($,.STERADIAN.)
SOLID_ANGLE_UNIT()
);
#32319=SHAPE_DEFINITION_REPRESENTATION(#32334,#32366);
#32334=PRODUCT_DEFINITION_SHAPE('',$,#32382);
#32366=SHAPE_REPRESENTATION('',(#14204),#32299);
#32376=PRODUCT_DEFINITION_CONTEXT('part definition',#32423,'design');
#32382=PRODUCT_DEFINITION('2026-10-25-00-35-16-655',
'05_Inner_Tube_2sq_x_3-16_Lock_Holes',#32397,#32376);
#32397=PRODUCT_DEFINITION_FORMATION('',$,#32430);
#32423=APPLICATION_CONTEXT(
'Core Data for Automotive Mechanical Design Process');
#32424=PRODUCT_CONTEXT('part definition',#32423,'mechanical');
#32430=PRODUCT('2026-10-25-00-35-16-655',
'05_Inner_Tube_2sq_x_3-16_Lock_Holes',$,(#32424));
#32482=COLOUR_RGB('Light Blue',0.38,0.62,0.78);
#32483=FILL_AREA_STYLE_COLOUR('',#32482);
#32484=FILL_AREA_STYLE('',(#32483));
#32485=SURFACE_STYLE_FILL_AREA(#32484);
#32486=SURFACE_SIDE_STYLE('',(#32485));
#32487=SURFACE_STYLE_USAGE(.BOTH.,#32486);
#32488=PRESENTATION_STYLE_ASSIGNMENT((#32487));
ENDSEC;
END-ISO-10303-21;
